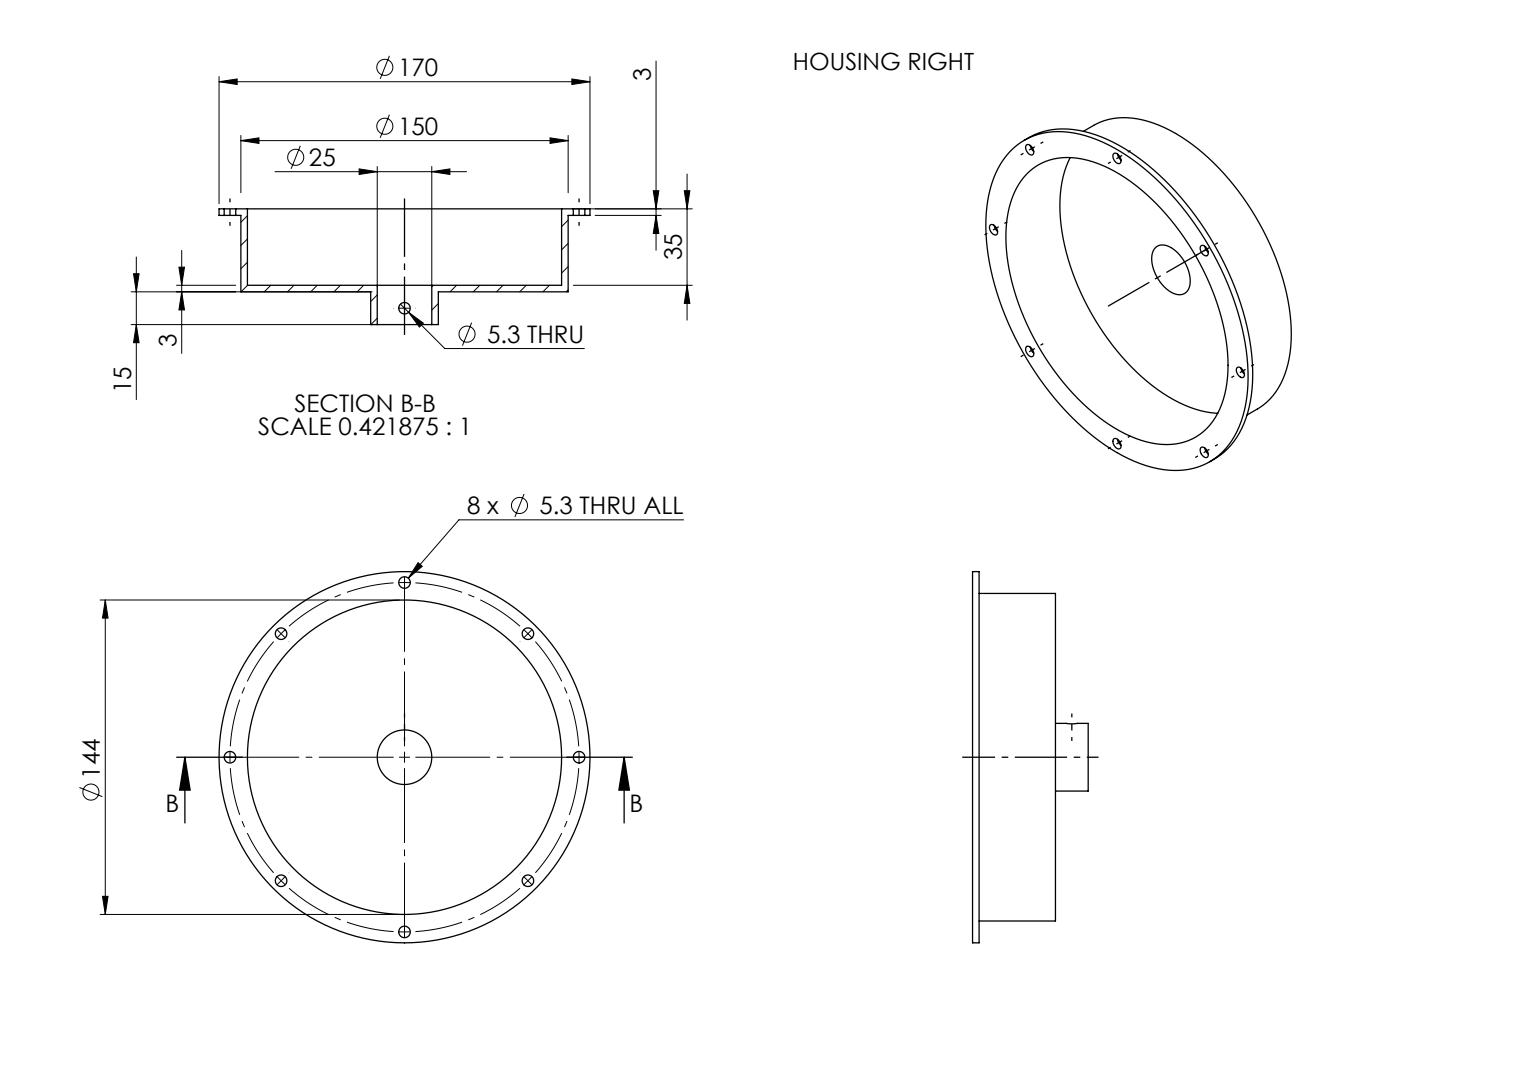
ISO-10303-21;
HEADER;
FILE_DESCRIPTION (('STEP AP214'),
    '1' );
FILE_NAME ('housing right.step',
    '2026-10-08T08:02:49',
    ( '' ),
    ( '' ),
    'SwSTEP 2.0',
    'SolidWorks 2026',
    '' );
FILE_SCHEMA (( 'AUTOMOTIVE_DESIGN' ));
ENDSEC;

DATA;
#5=FACE_OUTER_BOUND ( 'NONE', #24544, .T. ) ;
#96=VERTEX_POINT ( 'NONE', #35469 ) ;
#191=CARTESIAN_POINT ( 'NONE',  ( 52.60669624972128844, 15.41611702489417723, 1.616806307337775861 ) ) ;
#231=ORIENTED_EDGE ( 'NONE', *, *, #52615, .T. ) ;
#243=VERTEX_POINT ( 'NONE', #51378 ) ;
#255=ORIENTED_EDGE ( 'NONE', *, *, #39405, .T. ) ;
#274=COLOUR_RGB ( '', 0.66274510, 0.83137255, 0.94901961) ;
#323=DIRECTION ( 'NONE',  ( -1.000000000000000000, -5.380183451256670742E-17, 1.298891185607911324E-16 ) ) ;
#362=SHAPE_REPRESENTATION ( 'housing right', ( #14677 ), #14881 ) ;
#449=AXIS2_PLACEMENT_3D ( 'NONE', #23041, #9232, #46861 ) ;
#451=EDGE_CURVE ( 'NONE', #48858, #40875, #52468, .T. ) ;
#522=FACE_OUTER_BOUND ( 'NONE', #7239, .T. ) ;
#540=CARTESIAN_POINT ( 'NONE',  ( 52.25260954720639006, 15.37154784856826772, -1.995153943981983202 ) ) ;
#572=CARTESIAN_POINT ( 'NONE',  ( 5.000000000000007994, -58.44237546506767700, -54.69470952477997372 ) ) ;
#620=ORIENTED_EDGE ( 'NONE', *, *, #5146, .T. ) ;
#650=AXIS2_PLACEMENT_3D ( 'NONE', #4623, #9354, #47896 ) ;
#673=CARTESIAN_POINT ( 'NONE',  ( 8.000000000000007105, -56.56854249492331377, -56.56854249492430142 ) ) ;
#689=AXIS2_PLACEMENT_3D ( 'NONE', #15589, #28433, #47560 ) ;
#696=DIRECTION ( 'NONE',  ( -1.000000000000000000, -1.836909530733580185E-16, 1.836909530733574022E-16 ) ) ;
#702=EDGE_LOOP ( 'NONE', ( #10491, #19240, #32643, #32157 ) ) ;
#735=CIRCLE ( 'NONE', #51752, 2.649999999999997691 ) ;
#816=DIRECTION ( 'NONE',  ( 0.000000000000000000, 0.7071067811865527908, -0.7071067811865421326 ) ) ;
#915=AXIS2_PLACEMENT_3D ( 'NONE', #38595, #48285, #43928 ) ;
#936=CARTESIAN_POINT ( 'NONE',  ( 4.999999999999997335, 9.184547653667864935E-16, -9.629649721936170507E-32 ) ) ;
#958=DIRECTION ( 'NONE',  ( 0.000000000000000000, -0.7071067811865487940, 0.7071067811865461294 ) ) ;
#1011=ORIENTED_EDGE ( 'NONE', *, *, #3651, .F. ) ;
#1013=CARTESIAN_POINT ( 'NONE',  ( 50.50000000000000000, 0.000000000000000000, -2.649999999999992806 ) ) ;
#1079=EDGE_CURVE ( 'NONE', #57986, #43044, #10426, .T. ) ;
#1087=EDGE_LOOP ( 'NONE', ( #1602, #31859, #25371, #6168 ) ) ;
#1113=FACE_OUTER_BOUND ( 'NONE', #4513, .T. ) ;
#1258=CARTESIAN_POINT ( 'NONE',  ( 43.00000000000000000, -15.49999999999999645, -2.995852231480067093E-16 ) ) ;
#1274=DIRECTION ( 'NONE',  ( -1.000000000000000000, -1.836909530733573776E-16, 1.925929944387235853E-32 ) ) ;
#1387=DIRECTION ( 'NONE',  ( 0.000000000000000000, 0.000000000000000000, 1.000000000000000000 ) ) ;
#1485=ORIENTED_EDGE ( 'NONE', *, *, #15585, .F. ) ;
#1568=CARTESIAN_POINT ( 'NONE',  ( 52.88125656235560967, 12.44562621623030374, 1.175754242111713532 ) ) ;
#1596=FACE_BOUND ( 'NONE', #57316, .T. ) ;
#1602=ORIENTED_EDGE ( 'NONE', *, *, #33800, .T. ) ;
#1605=ORIENTED_EDGE ( 'NONE', *, *, #37368, .F. ) ;
#1646=EDGE_CURVE ( 'NONE', #14994, #48858, #28079, .T. ) ;
#1654=DIRECTION ( 'NONE',  ( -1.000000000000000000, -3.673819061467147552E-16, 1.925929944387235306E-32 ) ) ;
#1658=AXIS2_PLACEMENT_3D ( 'NONE', #1806, #16240, #49131 ) ;
#1757=CIRCLE ( 'NONE', #29764, 2.649999999999999467 ) ;
#1773=DIRECTION ( 'NONE',  ( -1.000000000000000000, -1.836909530733573776E-16, 1.925929944387235853E-32 ) ) ;
#1778=AXIS2_PLACEMENT_3D ( 'NONE', #20254, #15546, #816 ) ;
#1806=CARTESIAN_POINT ( 'NONE',  ( 5.000000000000007994, -56.56854249492410958, 56.56854249492351983 ) ) ;
#1810=VECTOR ( 'NONE', #7131, 1000.000000000000000 ) ;
#1818=FILL_AREA_STYLE_COLOUR ( '', #25853 ) ;
#1858=VERTEX_POINT ( 'NONE', #34439 ) ;
#1883=CARTESIAN_POINT ( 'NONE',  ( 52.61790645059762284, 12.39576633866792044, -1.629651744153580939 ) ) ;
#1887=VERTEX_POINT ( 'NONE', #36294 ) ;
#1938=VECTOR ( 'NONE', #21205, 1000.000000000000000 ) ;
#1939=CARTESIAN_POINT ( 'NONE',  ( 49.80403646751975799, 12.23154873426529399, 2.580195994037977059 ) ) ;
#2014=LINE ( 'NONE', #30525, #29451 ) ;
#2018=ORIENTED_EDGE ( 'NONE', *, *, #8269, .F. ) ;
#2024=CYLINDRICAL_SURFACE ( 'NONE', #46927, 2.649999999999992806 ) ;
#2160=AXIS2_PLACEMENT_3D ( 'NONE', #3680, #4593, #22815 ) ;
#2183=CARTESIAN_POINT ( 'NONE',  ( 51.83055647397077337, 12.28729589684768264, 2.298227778111301856 ) ) ;
#2186=ORIENTED_EDGE ( 'NONE', *, *, #37368, .T. ) ;
#2360=EDGE_CURVE ( 'NONE', #6447, #24288, #28038, .T. ) ;
#2369=FACE_OUTER_BOUND ( 'NONE', #43922, .T. ) ;
#2380=AXIS2_PLACEMENT_3D ( 'NONE', #47153, #47762, #5118 ) ;
#2435=( NAMED_UNIT ( * ) PLANE_ANGLE_UNIT ( ) SI_UNIT ( $, .RADIAN. ) );
#2488=DIRECTION ( 'NONE',  ( -1.000000000000000000, -3.673819061467147552E-16, 1.925929944387235306E-32 ) ) ;
#2499=CARTESIAN_POINT ( 'NONE',  ( 4.999999999999986677, 56.56854249492450037, -56.56854249492312192 ) ) ;
#2514=CARTESIAN_POINT ( 'NONE',  ( 5.000000000000010658, -72.00000000000002842, 8.817456953860946444E-15 ) ) ;
#2520=DIRECTION ( 'NONE',  ( 0.000000000000000000, 0.000000000000000000, -1.000000000000000000 ) ) ;
#2558=CARTESIAN_POINT ( 'NONE',  ( 50.50000000000000000, 12.21587082446438011, -2.649999999999992806 ) ) ;
#2661=CARTESIAN_POINT ( 'NONE',  ( 7.999999999999981348, 85.00000000000001421, 1.040949779275250495E-14 ) ) ;
#2744=SHAPE_REPRESENTATION_RELATIONSHIP ( 'NONE' , 'NONE' ,  #362, #34065 ) ;
#2748=CARTESIAN_POINT ( 'NONE',  ( 5.000000000000007994, -54.69470952477976056, 58.44237546506787595 ) ) ;
#2759=APPLICATION_CONTEXT ( 'automotive_design' ) ;
#2822=AXIS2_PLACEMENT_3D ( 'NONE', #46688, #22564, #41688 ) ;
#2939=CIRCLE ( 'NONE', #47947, 72.00000000000002842 ) ;
#2960=DIRECTION ( 'NONE',  ( -1.000000000000000000, -1.836909530733580185E-16, 1.836909530733574022E-16 ) ) ;
#3095=ORIENTED_EDGE ( 'NONE', *, *, #9104, .T. ) ;
#3162=ORIENTED_EDGE ( 'NONE', *, *, #6685, .T. ) ;
#3253=CARTESIAN_POINT ( 'NONE',  ( 7.999999999999986677, 56.56854249492371878, 56.56854249492391062 ) ) ;
#3375=DIRECTION ( 'NONE',  ( -1.850371707708593823E-16, 1.000000000000000000, 0.000000000000000000 ) ) ;
#3377=EDGE_LOOP ( 'NONE', ( #255, #7217 ) ) ;
#3435=CARTESIAN_POINT ( 'NONE',  ( 7.999999999999996447, -2.778489794828638662E-13, 80.00000000000001421 ) ) ;
#3442=ORIENTED_EDGE ( 'NONE', *, *, #8024, .T. ) ;
#3459=EDGE_CURVE ( 'NONE', #1887, #50598, #34882, .T. ) ;
#3517=ORIENTED_EDGE ( 'NONE', *, *, #21854, .T. ) ;
#3543=DIRECTION ( 'NONE',  ( 1.000000000000000000, 1.836909530733573776E-16, -1.925929944387235853E-32 ) ) ;
#3646=CYLINDRICAL_SURFACE ( 'NONE', #22822, 2.649999999999992806 ) ;
#3651=EDGE_CURVE ( 'NONE', #25227, #26701, #35913, .T. ) ;
#3663=SURFACE_STYLE_FILL_AREA ( #20946 ) ;
#3680=CARTESIAN_POINT ( 'NONE',  ( 50.50000000000000000, 0.000000000000000000, 0.000000000000000000 ) ) ;
#3688=ORIENTED_EDGE ( 'NONE', *, *, #12608, .T. ) ;
#3750=CARTESIAN_POINT ( 'NONE',  ( 5.000000000000007994, -56.56854249492331377, -56.56854249492430142 ) ) ;
#3759=CARTESIAN_POINT ( 'NONE',  ( 0.000000000000000000, 0.000000000000000000, 0.000000000000000000 ) ) ;
#3771=PRODUCT_DEFINITION ( 'UNKNOWN', '', #29877, #38625 ) ;
#3868=EDGE_CURVE ( 'NONE', #59695, #9789, #28867, .T. ) ;
#3988=DIRECTION ( 'NONE',  ( 1.000000000000000000, 1.836909530733573776E-16, -1.925929944387235853E-32 ) ) ;
#4013=ORIENTED_EDGE ( 'NONE', *, *, #28082, .F. ) ;
#4029=CYLINDRICAL_SURFACE ( 'NONE', #41805, 2.649999999999992806 ) ;
#4130=CARTESIAN_POINT ( 'NONE',  ( 4.999999999999997335, 9.184547653667862963E-16, -9.629649721936174886E-32 ) ) ;
#4147=DIRECTION ( 'NONE',  ( 0.000000000000000000, 0.000000000000000000, 1.000000000000000000 ) ) ;
#4151=ORIENTED_EDGE ( 'NONE', *, *, #33324, .F. ) ;
#4178=VERTEX_POINT ( 'NONE', #46032 ) ;
#4336=CARTESIAN_POINT ( 'NONE',  ( 48.39278666958532682, 15.41618682757451353, 1.616172141987365363 ) ) ;
#4381=CYLINDRICAL_SURFACE ( 'NONE', #50819, 75.00000000000001421 ) ;
#4513=EDGE_LOOP ( 'NONE', ( #27565, #49130, #52774, #5751 ) ) ;
#4525=FILL_AREA_STYLE ('',( #27429 ) ) ;
#4593=DIRECTION ( 'NONE',  ( -0.000000000000000000, -1.000000000000000000, -0.000000000000000000 ) ) ;
#4602=AXIS2_PLACEMENT_3D ( 'NONE', #19390, #61048, #61651 ) ;
#4623=CARTESIAN_POINT ( 'NONE',  ( 4.999999999999983125, 80.00000000000001421, -3.562970397116383044E-32 ) ) ;
#4633=CARTESIAN_POINT ( 'NONE',  ( 4.999999999999997335, 8.388739760877188892E-13, -80.00000000000001421 ) ) ;
#4691=AXIS2_PLACEMENT_3D ( 'NONE', #16594, #60110, #25989 ) ;
#4729=DIRECTION ( 'NONE',  ( 1.836766033387207149E-16, -1.000000000000000000, 0.000000000000000000 ) ) ;
#4788=AXIS2_PLACEMENT_3D ( 'NONE', #11876, #22481, #36916 ) ;
#4875=VERTEX_POINT ( 'NONE', #35777 ) ;
#4906=CIRCLE ( 'NONE', #24969, 2.649999999999997691 ) ;
#4930=CARTESIAN_POINT ( 'NONE',  ( 52.60613790598473116, 15.41603472375467909, -1.617730826299683899 ) ) ;
#4957=DIRECTION ( 'NONE',  ( -1.000000000000000000, -1.836909530733554547E-16, -1.836909530733573529E-16 ) ) ;
#5062=EDGE_LOOP ( 'NONE', ( #29514, #1605 ) ) ;
#5118=DIRECTION ( 'NONE',  ( 0.000000000000000000, 0.7071067811865527908, -0.7071067811865421326 ) ) ;
#5129=EDGE_CURVE ( 'NONE', #55350, #25443, #29738, .T. ) ;
#5146=EDGE_CURVE ( 'NONE', #48858, #14994, #26953, .T. ) ;
#5265=FACE_OUTER_BOUND ( 'NONE', #41410, .T. ) ;
#5329=CIRCLE ( 'NONE', #54330, 85.00000000000001421 ) ;
#5399=CARTESIAN_POINT ( 'NONE',  ( 7.999999999999996447, 8.394250489469390599E-13, -80.00000000000001421 ) ) ;
#5405=ORIENTED_EDGE ( 'NONE', *, *, #2360, .T. ) ;
#5468=AXIS2_PLACEMENT_3D ( 'NONE', #18420, #23729, #23419 ) ;
#5523=DIRECTION ( 'NONE',  ( -1.000000000000000000, -1.836909530733580185E-16, 1.836909530733574022E-16 ) ) ;
#5527=DIRECTION ( 'NONE',  ( 0.000000000000000000, -1.000000000000000000, 0.000000000000000000 ) ) ;
#5536=CARTESIAN_POINT ( 'NONE',  ( 52.88193763142881210, 15.45628894957374655, -1.174165929033795353 ) ) ;
#5751=ORIENTED_EDGE ( 'NONE', *, *, #6356, .T. ) ;
#5912=ORIENTED_EDGE ( 'NONE', *, *, #55151, .T. ) ;
#5918=ORIENTED_EDGE ( 'NONE', *, *, #2360, .F. ) ;
#5933=EDGE_LOOP ( 'NONE', ( #25583, #3095, #57007, #56092 ) ) ;
#5945=CARTESIAN_POINT ( 'NONE',  ( 52.49662775218939714, 12.37736723654698068, 1.751076765323000828 ) ) ;
#6168=ORIENTED_EDGE ( 'NONE', *, *, #45409, .F. ) ;
#6189=( NAMED_UNIT ( * ) SI_UNIT ( $, .STERADIAN. ) SOLID_ANGLE_UNIT ( ) );
#6210=EDGE_CURVE ( 'NONE', #50555, #49238, #25827, .T. ) ;
#6259=CARTESIAN_POINT ( 'NONE',  ( 58.00000000000000000, 15.50000000000000888, 1.598617315530390651E-15 ) ) ;
#6262=EDGE_CURVE ( 'NONE', #29773, #12923, #17251, .T. ) ;
#6335=LINE ( 'NONE', #54266, #37437 ) ;
#6356=EDGE_CURVE ( 'NONE', #9789, #59695, #14849, .T. ) ;
#6405=CARTESIAN_POINT ( 'NONE',  ( 39.99999999999998579, 72.00000000000004263, -4.333342374871279794E-31 ) ) ;
#6447=VERTEX_POINT ( 'NONE', #17435 ) ;
#6452=ORIENTED_EDGE ( 'NONE', *, *, #54819, .T. ) ;
#6535=ORIENTED_EDGE ( 'NONE', *, *, #18753, .T. ) ;
#6559=CARTESIAN_POINT ( 'NONE',  ( 51.18761205055119490, 12.23403309190988075, -2.565078866171123906 ) ) ;
#6561=EDGE_CURVE ( 'NONE', #16220, #6447, #22842, .T. ) ;
#6604=ORIENTED_EDGE ( 'NONE', *, *, #44026, .T. ) ;
#6663=CARTESIAN_POINT ( 'NONE',  ( 7.999999999999996447, -2.650000000000270806, 80.00000000000000000 ) ) ;
#6685=EDGE_CURVE ( 'NONE', #8457, #243, #58819, .T. ) ;
#6752=AXIS2_PLACEMENT_3D ( 'NONE', #21935, #59825, #26941 ) ;
#6776=ORIENTED_EDGE ( 'NONE', *, *, #49614, .F. ) ;
#6792=ORIENTED_EDGE ( 'NONE', *, *, #18019, .T. ) ;
#6906=CIRCLE ( 'NONE', #31942, 2.649999999999997691 ) ;
#6910=ADVANCED_FACE ( 'NONE', ( #28217 ), #4381, .T. ) ;
#7103=EDGE_LOOP ( 'NONE', ( #32035, #49413, #2186, #46245 ) ) ;
#7131=DIRECTION ( 'NONE',  ( -1.000000000000000000, -3.135800716341471541E-16, -1.298891185607920445E-16 ) ) ;
#7166=CIRCLE ( 'NONE', #44250, 75.00000000000001421 ) ;
#7217=ORIENTED_EDGE ( 'NONE', *, *, #9358, .T. ) ;
#7239=EDGE_LOOP ( 'NONE', ( #4013, #45371, #9473, #45138, #17668, #60804, #13702 ) ) ;
#7248=ORIENTED_EDGE ( 'NONE', *, *, #9104, .F. ) ;
#7252=AXIS2_PLACEMENT_3D ( 'NONE', #46444, #18538, #41751 ) ;
#7318=FACE_OUTER_BOUND ( 'NONE', #43411, .T. ) ;
#7362=EDGE_LOOP ( 'NONE', ( #28161, #35366 ) ) ;
#7366=CARTESIAN_POINT ( 'NONE',  ( 4.999999999999997335, 9.184547653667864935E-16, -9.629649721936170507E-32 ) ) ;
#7418=CARTESIAN_POINT ( 'NONE',  ( 8.000000000000007105, -56.56854249492331377, -56.56854249492430142 ) ) ;
#7424=ORIENTED_EDGE ( 'NONE', *, *, #9041, .F. ) ;
#7460=VECTOR ( 'NONE', #50221, 1000.000000000000000 ) ;
#7471=CARTESIAN_POINT ( 'NONE',  ( 5.000000000000013323, -85.00000000000001421, -9.629649721936174886E-32 ) ) ;
#7492=VECTOR ( 'NONE', #43754, 1000.000000000000000 ) ;
#7504=ORIENTED_EDGE ( 'NONE', *, *, #22869, .F. ) ;
#7537=FACE_OUTER_BOUND ( 'NONE', #45126, .T. ) ;
#7552=ORIENTED_EDGE ( 'NONE', *, *, #43108, .T. ) ;
#7686=DIRECTION ( 'NONE',  ( -1.836909530733573776E-16, 1.000000000000000000, 0.000000000000000000 ) ) ;
#7765=PRODUCT ( 'housing right', 'housing right', '', ( #12722 ) ) ;
#7842=DIRECTION ( 'NONE',  ( 1.000000000000000000, 1.836909530733573776E-16, -1.925929944387235853E-32 ) ) ;
#8024=EDGE_CURVE ( 'NONE', #25443, #22251, #31564, .T. ) ;
#8185=CARTESIAN_POINT ( 'NONE',  ( 50.15117465005047137, 12.21965674021488368, -2.632719331364402393 ) ) ;
#8192=ORIENTED_EDGE ( 'NONE', *, *, #38584, .F. ) ;
#8232=ORIENTED_EDGE ( 'NONE', *, *, #54819, .F. ) ;
#8233=DIRECTION ( 'NONE',  ( -1.000000000000000000, -5.380183451256670742E-17, 1.298891185607911324E-16 ) ) ;
#8259=ORIENTED_EDGE ( 'NONE', *, *, #9041, .T. ) ;
#8269=EDGE_CURVE ( 'NONE', #29773, #54373, #53933, .T. ) ;
#8444=DIRECTION ( 'NONE',  ( 0.000000000000000000, 1.000000000000000000, 0.000000000000000000 ) ) ;
#8457=VERTEX_POINT ( 'NONE', #42351 ) ;
#8487=FACE_OUTER_BOUND ( 'NONE', #10114, .T. ) ;
#8569=AXIS2_PLACEMENT_3D ( 'NONE', #936, #23828, #33241 ) ;
#8609=AXIS2_PLACEMENT_3D ( 'NONE', #29297, #48408, #14919 ) ;
#8680=CARTESIAN_POINT ( 'NONE',  ( 52.25008115675156972, 15.37124894287441279, 1.997531998838311784 ) ) ;
#8691=DIRECTION ( 'NONE',  ( 1.000000000000000000, 1.836909530733573776E-16, -1.925929944387235853E-32 ) ) ;
#8716=CARTESIAN_POINT ( 'NONE',  ( 4.999999999999997335, 8.388739760877188892E-13, -80.00000000000001421 ) ) ;
#8771=CARTESIAN_POINT ( 'NONE',  ( 8.000000000000007105, -58.44237546506767700, -54.69470952477997372 ) ) ;
#8776=AXIS2_PLACEMENT_3D ( 'NONE', #7366, #21488, #59694 ) ;
#8848=CYLINDRICAL_SURFACE ( 'NONE', #35618, 85.00000000000001421 ) ;
#8861=EDGE_CURVE ( 'NONE', #12452, #23359, #2014, .T. ) ;
#9026=CARTESIAN_POINT ( 'NONE',  ( 53.01412262506746487, 15.47721078833569841, -0.8552660025069994676 ) ) ;
#9041=EDGE_CURVE ( 'NONE', #15197, #37408, #42738, .T. ) ;
#9065=CARTESIAN_POINT ( 'NONE',  ( 48.74902663329513786, 15.37135949308304816, 1.996608280103705058 ) ) ;
#9104=EDGE_CURVE ( 'NONE', #22095, #22251, #38658, .T. ) ;
#9135=ORIENTED_EDGE ( 'NONE', *, *, #48508, .F. ) ;
#9145=CARTESIAN_POINT ( 'NONE',  ( 50.50000000000000000, 15.27178771460631168, -2.649999999999992806 ) ) ;
#9196=DIRECTION ( 'NONE',  ( 0.000000000000000000, -1.047444401652941269E-14, 1.000000000000000000 ) ) ;
#9222=EDGE_LOOP ( 'NONE', ( #6535, #46586 ) ) ;
#9232=DIRECTION ( 'NONE',  ( 1.000000000000000000, 1.836909530733573776E-16, -1.925929944387235853E-32 ) ) ;
#9295=ORIENTED_EDGE ( 'NONE', *, *, #33396, .T. ) ;
#9302=CARTESIAN_POINT ( 'NONE',  ( 53.06470156691138129, 15.48560858660915507, 0.6891024955566218413 ) ) ;
#9314=CARTESIAN_POINT ( 'NONE',  ( 50.32467004767242713, 15.27178771460630635, -2.649999999999991918 ) ) ;
#9339=EDGE_CURVE ( 'NONE', #49193, #29142, #52340, .T. ) ;
#9354=DIRECTION ( 'NONE',  ( -1.000000000000000000, -0.000000000000000000, 1.925929944387235853E-32 ) ) ;
#9358=EDGE_CURVE ( 'NONE', #22596, #20457, #26502, .T. ) ;
#9367=ORIENTED_EDGE ( 'NONE', *, *, #22995, .F. ) ;
#9473=ORIENTED_EDGE ( 'NONE', *, *, #451, .T. ) ;
#9529=DIRECTION ( 'NONE',  ( 0.000000000000000000, 0.000000000000000000, -1.000000000000000000 ) ) ;
#9535=APPLICATION_CONTEXT ( 'automotive_design' ) ;
#9621=EDGE_LOOP ( 'NONE', ( #48967, #45953 ) ) ;
#9625=CARTESIAN_POINT ( 'NONE',  ( 50.15149541334723438, 15.27480702088406694, -2.632769263815124994 ) ) ;
#9720=FACE_BOUND ( 'NONE', #40678, .T. ) ;
#9789=VERTEX_POINT ( 'NONE', #43524 ) ;
#9848=EDGE_CURVE ( 'NONE', #26701, #25227, #25509, .T. ) ;
#9962=ORIENTED_EDGE ( 'NONE', *, *, #60027, .T. ) ;
#9966=CARTESIAN_POINT ( 'NONE',  ( 51.35572961735444153, 15.29490605596151553, -2.514040278272794637 ) ) ;
#9971=FACE_BOUND ( 'NONE', #15664, .T. ) ;
#9990=VERTEX_POINT ( 'NONE', #37206 ) ;
#9996=ORIENTED_EDGE ( 'NONE', *, *, #3868, .F. ) ;
#10003=ADVANCED_FACE ( 'NONE', ( #46598 ), #3646, .F. ) ;
#10114=EDGE_LOOP ( 'NONE', ( #1485, #33255, #6452, #29907 ) ) ;
#10122=CARTESIAN_POINT ( 'NONE',  ( 48.88249858120726543, 12.32166152761977429, 2.106239978570320304 ) ) ;
#10185=( NAMED_UNIT ( * ) PLANE_ANGLE_UNIT ( ) SI_UNIT ( $, .RADIAN. ) );
#10349=FACE_BOUND ( 'NONE', #25658, .T. ) ;
#10385=B_SPLINE_CURVE_WITH_KNOTS ( 'NONE', 3,
 ( #37601, #61357, #38524, #22865, #61061, #18474, #13793, #32897, #9065, #47288, #4336, #18795, #37921, #34132, #35058, #35368, #40086, #34434 ),
 .UNSPECIFIED., .F., .F.,
 ( 4, 2, 2, 2, 2, 2, 2, 2, 4 ),
 ( 0.008300350213780812239, 0.008819185130678563675, 0.009338020047576315111, 0.009856854964474064812, 0.01037568988137181625, 0.01089452479826956768, 0.01141335971516731912, 0.01193219463206507056, 0.01245102954896282026 ),
 .UNSPECIFIED. ) ;
#10426=LINE ( 'NONE', #24830, #18072 ) ;
#10491=ORIENTED_EDGE ( 'NONE', *, *, #1079, .F. ) ;
#10532=CARTESIAN_POINT ( 'NONE',  ( 40.00000000000000000, 7.347638122934295104E-15, -7.703719777548943412E-31 ) ) ;
#10550=ADVANCED_FACE ( 'NONE', ( #61064 ), #53888, .T. ) ;
#10568=CARTESIAN_POINT ( 'NONE',  ( 4.999999999999986677, 54.69470952478017267, -58.44237546506749936 ) ) ;
#10979=CARTESIAN_POINT ( 'NONE',  ( 4.999999999999998224, -2.649999999999161471, -80.00000000000004263 ) ) ;
#10987=EDGE_LOOP ( 'NONE', ( #14158, #38902, #31865, #59387 ) ) ;
#11005=CARTESIAN_POINT ( 'NONE',  ( 51.35620144615297988, 12.24479674684753761, -2.513874600954978167 ) ) ;
#11054=CLOSED_SHELL ( 'NONE', ( #16134, #10550, #43383, #44525, #10003, #33207, #22022, #53580, #21743, #61635, #57359, #12192, #56573, #6910, #14160, #21274, #61922, #39300, #56281, #22127, #57051, #53773, #44022, #56991, #18338, #61290, #18801, #33471, #55309, #46488, #45799, #21069, #49011 ) ) ;
#11059=DIRECTION ( 'NONE',  ( -0.000000000000000000, -1.000000000000000000, -0.000000000000000000 ) ) ;
#11203=PLANE ( 'NONE',  #45538 ) ;
#11240=( LENGTH_UNIT ( ) NAMED_UNIT ( * ) SI_UNIT ( .MILLI., .METRE. ) );
#11292=ORIENTED_EDGE ( 'NONE', *, *, #22869, .T. ) ;
#11301=CARTESIAN_POINT ( 'NONE',  ( 53.14993166107466749, 12.49998551214889808, -0.1744414439710397502 ) ) ;
#11474=DIRECTION ( 'NONE',  ( 0.000000000000000000, 0.000000000000000000, 1.000000000000000000 ) ) ;
#11504=LINE ( 'NONE', #49703, #1938 ) ;
#11591=ORIENTED_EDGE ( 'NONE', *, *, #39069, .F. ) ;
#11764=CIRCLE ( 'NONE', #59771, 2.649999999999985700 ) ;
#11819=EDGE_LOOP ( 'NONE', ( #33452, #27207, #61717, #49182, #46180 ) ) ;
#11831=EDGE_CURVE ( 'NONE', #33073, #1887, #46628, .T. ) ;
#11848=EDGE_CURVE ( 'NONE', #49193, #29773, #27107, .T. ) ;
#11876=CARTESIAN_POINT ( 'NONE',  ( 4.999999999999983125, 80.00000000000001421, -3.562970397116383044E-32 ) ) ;
#11887=CARTESIAN_POINT ( 'NONE',  ( 5.000000000000007994, -54.69470952477895764, -58.44237546506863623 ) ) ;
#12002=CARTESIAN_POINT ( 'NONE',  ( 50.50000000000000000, 12.21587082446438011, -2.649999999999992806 ) ) ;
#12004=DIRECTION ( 'NONE',  ( -1.000000000000000000, -1.836909530733554547E-16, -1.836909530733573529E-16 ) ) ;
#12036=CARTESIAN_POINT ( 'NONE',  ( 4.999999999999986677, 56.56854249492371878, 56.56854249492391062 ) ) ;
#12040=LINE ( 'NONE', #12648, #7460 ) ;
#12110=SHAPE_DEFINITION_REPRESENTATION ( #50273, #362 ) ;
#12192=ADVANCED_FACE ( 'NONE', ( #2369 ), #21809, .F. ) ;
#12247=LINE ( 'NONE', #40159, #30933 ) ;
#12428=AXIS2_PLACEMENT_3D ( 'NONE', #25100, #1274, #39536 ) ;
#12452=VERTEX_POINT ( 'NONE', #6663 ) ;
#12520=DIRECTION ( 'NONE',  ( 0.000000000000000000, 0.7071067811865395791, 0.7071067811865553443 ) ) ;
#12608=EDGE_CURVE ( 'NONE', #61948, #59796, #34720, .T. ) ;
#12648=CARTESIAN_POINT ( 'NONE',  ( 4.999999999999986677, 58.44237546506882808, -54.69470952477875869 ) ) ;
#12653=ORIENTED_EDGE ( 'NONE', *, *, #54361, .T. ) ;
#12681=DIRECTION ( 'NONE',  ( 1.850371707708593823E-16, -1.000000000000000000, 0.000000000000000000 ) ) ;
#12722=PRODUCT_CONTEXT ( 'NONE', #9535, 'mechanical' ) ;
#12806=DIRECTION ( 'NONE',  ( -1.000000000000000000, -1.836909530733573776E-16, 1.103352205049209901E-32 ) ) ;
#12834=CARTESIAN_POINT ( 'NONE',  ( 4.999999999999986677, 56.56854249492450037, -56.56854249492312192 ) ) ;
#12880=CARTESIAN_POINT ( 'NONE',  ( 43.00000000000000000, 5.682605120120046040E-15, -2.995852231480065614E-16 ) ) ;
#12895=CARTESIAN_POINT ( 'NONE',  ( 4.999999999999997335, 9.184547653667864935E-16, -9.629649721936170507E-32 ) ) ;
#12923=VERTEX_POINT ( 'NONE', #60160 ) ;
#12933=CYLINDRICAL_SURFACE ( 'NONE', #38608, 2.649999999999992806 ) ;
#12952=DIRECTION ( 'NONE',  ( 0.000000000000000000, 0.000000000000000000, -1.000000000000000000 ) ) ;
#13009=DIRECTION ( 'NONE',  ( 0.000000000000000000, -0.7071067811865461294, -0.7071067811865487940 ) ) ;
#13023=CARTESIAN_POINT ( 'NONE',  ( 8.000000000000012434, -80.00000000000001421, 2.649999999999992806 ) ) ;
#13040=EDGE_LOOP ( 'NONE', ( #29972, #17063 ) ) ;
#13095=ORIENTED_EDGE ( 'NONE', *, *, #28488, .T. ) ;
#13104=( NAMED_UNIT ( * ) PLANE_ANGLE_UNIT ( ) SI_UNIT ( $, .RADIAN. ) );
#13136=ORIENTED_EDGE ( 'NONE', *, *, #31544, .T. ) ;
#13366=CARTESIAN_POINT ( 'NONE',  ( 7.999999999999996447, -2.778489794828638662E-13, 80.00000000000001421 ) ) ;
#13415=LINE ( 'NONE', #22496, #19236 ) ;
#13477=AXIS2_PLACEMENT_3D ( 'NONE', #12834, #13760, #12520 ) ;
#13702=ORIENTED_EDGE ( 'NONE', *, *, #6262, .T. ) ;
#13760=DIRECTION ( 'NONE',  ( -1.000000000000000000, -5.380183451256491399E-17, -1.298891185607892835E-16 ) ) ;
#13788=CIRCLE ( 'NONE', #48771, 2.649999999999985700 ) ;
#13793=CARTESIAN_POINT ( 'NONE',  ( 49.17116576101606995, 15.32881676279135874, 2.299327193150783266 ) ) ;
#13822=DIRECTION ( 'NONE',  ( 1.000000000000000000, 0.000000000000000000, 0.000000000000000000 ) ) ;
#13900=VERTEX_POINT ( 'NONE', #2748 ) ;
#13988=CARTESIAN_POINT ( 'NONE',  ( 58.00000000000000000, 0.000000000000000000, 12.50000000000000000 ) ) ;
#14062=CARTESIAN_POINT ( 'NONE',  ( 53.14999999999999858, 15.50000000000000711, 1.598617295522242905E-15 ) ) ;
#14081=CYLINDRICAL_SURFACE ( 'NONE', #650, 2.649999999999992806 ) ;
#14136=ORIENTED_EDGE ( 'NONE', *, *, #54361, .F. ) ;
#14139=FACE_BOUND ( 'NONE', #43742, .T. ) ;
#14158=ORIENTED_EDGE ( 'NONE', *, *, #44026, .F. ) ;
#14160=ADVANCED_FACE ( 'NONE', ( #35215 ), #57746, .T. ) ;
#14198=ORIENTED_EDGE ( 'NONE', *, *, #61572, .F. ) ;
#14236=LINE ( 'NONE', #18937, #28561 ) ;
#14290=DIRECTION ( 'NONE',  ( -1.000000000000000000, -1.836909530733573776E-16, 1.925929944387235853E-32 ) ) ;
#14309=EDGE_LOOP ( 'NONE', ( #7424, #50025, #6792, #52169 ) ) ;
#14338=CARTESIAN_POINT ( 'NONE',  ( 51.35430322215398746, 15.29482815186059774, 2.514508868274447639 ) ) ;
#14577=ORIENTED_EDGE ( 'NONE', *, *, #451, .F. ) ;
#14597=CARTESIAN_POINT ( 'NONE',  ( 58.00000000000000000, -15.49999999999999112, -2.995852231480068572E-16 ) ) ;
#14639=CARTESIAN_POINT ( 'NONE',  ( 43.00000000000000000, 15.50000000000000533, 1.598617315530390848E-15 ) ) ;
#14654=EDGE_LOOP ( 'NONE', ( #1011, #59641, #27688, #6776 ) ) ;
#14674=CARTESIAN_POINT ( 'NONE',  ( 53.15000000000000568, 15.50000000000000711, -0.1732459626436144429 ) ) ;
#14677=AXIS2_PLACEMENT_3D ( 'NONE', #3759, #61387, #13822 ) ;
#14724=VERTEX_POINT ( 'NONE', #18187 ) ;
#14824=VECTOR ( 'NONE', #46380, 1000.000000000000000 ) ;
#14849=CIRCLE ( 'NONE', #59853, 2.649999999999997691 ) ;
#14881=( GEOMETRIC_REPRESENTATION_CONTEXT ( 3 ) GLOBAL_UNCERTAINTY_ASSIGNED_CONTEXT ( ( #48012 ) ) GLOBAL_UNIT_ASSIGNED_CONTEXT ( ( #11240, #2435, #6189 ) ) REPRESENTATION_CONTEXT ( 'NONE', 'WORKASPACE' ) );
#14919=DIRECTION ( 'NONE',  ( 0.000000000000000000, -0.7071067811865553443, 0.7071067811865395791 ) ) ;
#14969=CARTESIAN_POINT ( 'NONE',  ( 4.999999999999997335, -2.784000523420839360E-13, 80.00000000000001421 ) ) ;
#14987=AXIS2_PLACEMENT_3D ( 'NONE', #46493, #3543, #42125 ) ;
#14994=VERTEX_POINT ( 'NONE', #45705 ) ;
#15073=ORIENTED_EDGE ( 'NONE', *, *, #32108, .F. ) ;
#15197=VERTEX_POINT ( 'NONE', #32219 ) ;
#15397=CARTESIAN_POINT ( 'NONE',  ( 51.18991377541220800, 12.23415317001104086, 2.564509504438283294 ) ) ;
#15418=CARTESIAN_POINT ( 'NONE',  ( 4.999999999999986677, 56.56854249492450037, -56.56854249492312192 ) ) ;
#15444=CARTESIAN_POINT ( 'NONE',  ( 47.85015878647476484, 12.49996633727064932, 0.3510238927397298925 ) ) ;
#15462=CARTESIAN_POINT ( 'NONE',  ( 8.000000000000007105, -54.69470952477895764, -58.44237546506863623 ) ) ;
#15546=DIRECTION ( 'NONE',  ( -1.000000000000000000, -3.135800716341471541E-16, -1.298891185607920445E-16 ) ) ;
#15585=EDGE_CURVE ( 'NONE', #22596, #50555, #39020, .T. ) ;
#15589=CARTESIAN_POINT ( 'NONE',  ( 40.00000000000000000, 0.000000000000000000, 0.000000000000000000 ) ) ;
#15657=CIRCLE ( 'NONE', #4602, 15.50000000000000000 ) ;
#15664=EDGE_LOOP ( 'NONE', ( #30806, #31931 ) ) ;
#15704=CARTESIAN_POINT ( 'NONE',  ( 50.50000000000000000, 12.21587082446438011, 2.649999999999992806 ) ) ;
#15718=AXIS2_PLACEMENT_3D ( 'NONE', #22657, #43016, #61452 ) ;
#15757=CARTESIAN_POINT ( 'NONE',  ( 48.20159250628719150, 12.42985392437715220, 1.330251472907249433 ) ) ;
#15791=DIRECTION ( 'NONE',  ( -1.000000000000000000, -3.673819061467147552E-16, 1.925929944387235306E-32 ) ) ;
#15863=ORIENTED_EDGE ( 'NONE', *, *, #60454, .T. ) ;
#15904=FACE_BOUND ( 'NONE', #24389, .T. ) ;
#15995=DIRECTION ( 'NONE',  ( -1.000000000000000000, -1.836909530733573529E-16, 1.361838123766461297E-32 ) ) ;
#16012=CARTESIAN_POINT ( 'NONE',  ( 53.01364348093722612, 12.47163566169240845, -0.8566609489383912868 ) ) ;
#16128=DIRECTION ( 'NONE',  ( 0.000000000000000000, 0.000000000000000000, -1.000000000000000000 ) ) ;
#16131=EDGE_CURVE ( 'NONE', #55350, #22095, #7166, .T. ) ;
#16134=ADVANCED_FACE ( 'NONE', ( #17814 ), #42555, .F. ) ;
#16182=ORIENTED_EDGE ( 'NONE', *, *, #28199, .F. ) ;
#16220=VERTEX_POINT ( 'NONE', #43806 ) ;
#16240=DIRECTION ( 'NONE',  ( -1.000000000000000000, -3.135800716341489291E-16, 1.298891185607901956E-16 ) ) ;
#16271=ORIENTED_EDGE ( 'NONE', *, *, #11848, .F. ) ;
#16303=DIRECTION ( 'NONE',  ( 0.000000000000000000, 0.7071067811865382469, 0.7071067811865566766 ) ) ;
#16318=DIRECTION ( 'NONE',  ( -1.000000000000000000, -1.836909530733573776E-16, 1.925929944387235853E-32 ) ) ;
#16496=AXIS2_PLACEMENT_3D ( 'NONE', #38904, #23850, #32959 ) ;
#16538=DIRECTION ( 'NONE',  ( 0.000000000000000000, 0.7071067811865421326, 0.7071067811865527908 ) ) ;
#16581=B_SPLINE_CURVE_WITH_KNOTS ( 'NONE', 3,
 ( #20701, #29783, #39841, #6559, #11005, #58894, #40449, #30703, #49819, #1883, #35126, #16012, #58575, #16623, #11301, #30389, #54184, #59512, #58266, #1568, #53882, #48894, #5945, #26018, #25084, #2183, #44537, #44230, #15397, #54491, #49506, #15704 ),
 .UNSPECIFIED., .F., .F.,
 ( 4, 2, 2, 2, 2, 2, 2, 2, 2, 2, 2, 2, 2, 2, 2, 4 ),
 ( 0.000000000000000000, 0.0005192934025038106532, 0.001038586805007621306, 0.001557880207511431851, 0.002077173610015242613, 0.003115760415022862835, 0.003635053817526677066, 0.004154347220030491297, 0.004673640622534305095, 0.005192934025038119759, 0.005712227427541933557, 0.006231520830045749089, 0.006750814232549562886, 0.007270107635053377551, 0.007789401037557191348, 0.008308694440061006881 ),
 .UNSPECIFIED. ) ;
#16594=CARTESIAN_POINT ( 'NONE',  ( 4.999999999999997335, 9.184547653667864935E-16, -9.629649721936170507E-32 ) ) ;
#16623=CARTESIAN_POINT ( 'NONE',  ( 53.13300907242233251, 12.49636441417896116, -0.3467375140025887870 ) ) ;
#16704=CARTESIAN_POINT ( 'NONE',  ( 58.00000000000000000, 8.437969416220405915E-15, -2.995852231480068572E-16 ) ) ;
#16979=DIRECTION ( 'NONE',  ( -3.273063162220399693E-16, 1.000000000000000000, 1.047380211910527902E-14 ) ) ;
#17059=CARTESIAN_POINT ( 'NONE',  ( 4.999999999999997335, 9.184547653667862963E-16, -9.629649721936174886E-32 ) ) ;
#17063=ORIENTED_EDGE ( 'NONE', *, *, #6210, .F. ) ;
#17070=CYLINDRICAL_SURFACE ( 'NONE', #21765, 12.50000000000000000 ) ;
#17117=DIRECTION ( 'NONE',  ( 1.000000000000000000, 1.836909530733573776E-16, -1.925929944387235853E-32 ) ) ;
#17251=B_SPLINE_CURVE_WITH_KNOTS ( 'NONE', 3,
 ( #28436, #37562, #33787, #47876, #9966, #47253, #43817, #29067, #540, #38485, #4930, #38800, #5536, #9026, #24061, #57539, #14674, #14062 ),
 .UNSPECIFIED., .F., .F.,
 ( 4, 2, 2, 2, 2, 2, 2, 2, 4 ),
 ( 0.000000000000000000, 0.0005188972795902839106, 0.001037794559180567821, 0.001556691838770851623, 0.002075589118361135643, 0.002594486397951419662, 0.003113383677541703247, 0.003632280957131987266, 0.004151178236722271285 ),
 .UNSPECIFIED. ) ;
#17257=CARTESIAN_POINT ( 'NONE',  ( 8.000000000000012434, -80.00000000000001421, -2.147411887991766662E-31 ) ) ;
#17278=CARTESIAN_POINT ( 'NONE',  ( 43.00000000000000000, 0.000000000000000000, 0.000000000000000000 ) ) ;
#17389=DIRECTION ( 'NONE',  ( -1.000000000000000000, -1.836909530733573776E-16, 1.925929944387235853E-32 ) ) ;
#17423=( LENGTH_UNIT ( ) NAMED_UNIT ( * ) SI_UNIT ( .MILLI., .METRE. ) );
#17435=CARTESIAN_POINT ( 'NONE',  ( 7.999999999999986677, 54.69470952477936976, 58.44237546506825964 ) ) ;
#17575=AXIS2_PLACEMENT_3D ( 'NONE', #24916, #35244, #16128 ) ;
#17580=DIRECTION ( 'NONE',  ( -1.807003620809173399E-16, 1.000000000000000000, 0.000000000000000000 ) ) ;
#17650=ORIENTED_EDGE ( 'NONE', *, *, #38858, .T. ) ;
#17668=ORIENTED_EDGE ( 'NONE', *, *, #9339, .F. ) ;
#17737=DIRECTION ( 'NONE',  ( -1.000000000000000000, -3.135800716341489291E-16, 1.298891185607901956E-16 ) ) ;
#17742=CIRCLE ( 'NONE', #4691, 72.00000000000002842 ) ;
#17782=VECTOR ( 'NONE', #18110, 1000.000000000000000 ) ;
#17814=FACE_OUTER_BOUND ( 'NONE', #56413, .T. ) ;
#17874=EDGE_LOOP ( 'NONE', ( #17650, #53176 ) ) ;
#17887=AXIS2_PLACEMENT_3D ( 'NONE', #673, #28883, #19816 ) ;
#17947=EDGE_CURVE ( 'NONE', #22095, #55350, #61278, .T. ) ;
#17982=AXIS2_PLACEMENT_3D ( 'NONE', #22211, #41340, #51310 ) ;
#18007=DIRECTION ( 'NONE',  ( -1.000000000000000000, -5.380183451256670742E-17, 1.298891185607911324E-16 ) ) ;
#18019=EDGE_CURVE ( 'NONE', #96, #50941, #23854, .T. ) ;
#18072=VECTOR ( 'NONE', #696, 1000.000000000000000 ) ;
#18110=DIRECTION ( 'NONE',  ( -1.000000000000000000, -1.836909530733573776E-16, 1.925929944387235579E-32 ) ) ;
#18187=CARTESIAN_POINT ( 'NONE',  ( 50.50000000000000000, 12.21587082446438011, 2.649999999999992806 ) ) ;
#18198=FACE_OUTER_BOUND ( 'NONE', #10987, .T. ) ;
#18270=ORIENTED_EDGE ( 'NONE', *, *, #45409, .T. ) ;
#18338=ADVANCED_FACE ( 'NONE', ( #5265 ), #4029, .F. ) ;
#18365=CARTESIAN_POINT ( 'NONE',  ( 5.000000000000007994, -56.56854249492410958, 56.56854249492351983 ) ) ;
#18413=CARTESIAN_POINT ( 'NONE',  ( 53.01450034489953111, 15.47727011842658307, 0.8544031610831416268 ) ) ;
#18420=CARTESIAN_POINT ( 'NONE',  ( 7.999999999999996447, 1.469527624586858429E-15, -1.540743955509788245E-31 ) ) ;
#18422=CARTESIAN_POINT ( 'NONE',  ( 47.98575327796820744, 15.47722964620001385, -0.8550501376822413624 ) ) ;
#18474=CARTESIAN_POINT ( 'NONE',  ( 49.32574372153255382, 15.31603864467538934, 2.381899414255259639 ) ) ;
#18538=DIRECTION ( 'NONE',  ( 1.000000000000000000, 1.836909530733573776E-16, -1.925929944387235853E-32 ) ) ;
#18677=DIRECTION ( 'NONE',  ( 0.000000000000000000, 0.7071067811865500152, -0.7071067811865449082 ) ) ;
#18683=DIRECTION ( 'NONE',  ( -1.000000000000000000, -1.836909530733573776E-16, 2.465190328815655050E-32 ) ) ;
#18722=CARTESIAN_POINT ( 'NONE',  ( 51.82989359177101107, 15.32891900549394038, 2.298613371999423727 ) ) ;
#18753=EDGE_CURVE ( 'NONE', #18771, #44393, #32809, .T. ) ;
#18771=VERTEX_POINT ( 'NONE', #6405 ) ;
#18795=CARTESIAN_POINT ( 'NONE',  ( 48.20074816270739859, 15.44360797527890483, 1.328834602619866967 ) ) ;
#18801=ADVANCED_FACE ( 'NONE', ( #1113 ), #43772, .F. ) ;
#18879=VECTOR ( 'NONE', #30536, 1000.000000000000000 ) ;
#18937=CARTESIAN_POINT ( 'NONE',  ( 43.00000000000000000, 0.000000000000000000, 12.50000000000000000 ) ) ;
#18956=ORIENTED_EDGE ( 'NONE', *, *, #1646, .T. ) ;
#19022=ORIENTED_EDGE ( 'NONE', *, *, #56510, .T. ) ;
#19024=DIRECTION ( 'NONE',  ( -1.000000000000000000, -3.673819061467147552E-16, 1.925929944387235306E-32 ) ) ;
#19053=CARTESIAN_POINT ( 'NONE',  ( 48.19985924247141185, 15.44373933981895952, -1.327350711001176631 ) ) ;
#19155=VECTOR ( 'NONE', #46233, 1000.000000000000000 ) ;
#19227=EDGE_LOOP ( 'NONE', ( #23087, #47498, #19022, #27535, #28345, #56112, #14577 ) ) ;
#19236=VECTOR ( 'NONE', #8691, 1000.000000000000000 ) ;
#19240=ORIENTED_EDGE ( 'NONE', *, *, #25179, .F. ) ;
#19260=EDGE_CURVE ( 'NONE', #61948, #28137, #51354, .T. ) ;
#19370=FACE_BOUND ( 'NONE', #25814, .T. ) ;
#19390=CARTESIAN_POINT ( 'NONE',  ( 43.00000000000000000, 5.682605120120046040E-15, -2.995852231480065614E-16 ) ) ;
#19409=AXIS2_PLACEMENT_3D ( 'NONE', #36142, #50823, #12952 ) ;
#19660=CARTESIAN_POINT ( 'NONE',  ( 47.85000000000000853, 15.50000000000000711, 1.598617397282144235E-15 ) ) ;
#19683=DIRECTION ( 'NONE',  ( 1.000000000000000000, 1.836909530733573776E-16, -1.925929944387235853E-32 ) ) ;
#19816=DIRECTION ( 'NONE',  ( 0.000000000000000000, 0.7071067811865421326, 0.7071067811865527908 ) ) ;
#19848=DIRECTION ( 'NONE',  ( 0.000000000000000000, -0.7071067811865435759, -0.7071067811865514585 ) ) ;
#19877=CIRCLE ( 'NONE', #57848, 2.649999999999992806 ) ;
#19878=CARTESIAN_POINT ( 'NONE',  ( 5.000000000000007994, -58.44237546506844438, 54.69470952477915660 ) ) ;
#19920=DIRECTION ( 'NONE',  ( 0.000000000000000000, 0.000000000000000000, 1.000000000000000000 ) ) ;
#19944=CARTESIAN_POINT ( 'NONE',  ( 5.000000000000007994, -58.44237546506844438, 54.69470952477916370 ) ) ;
#20057=DIRECTION ( 'NONE',  ( 1.000000000000000000, 1.836909530733573776E-16, -1.925929944387235853E-32 ) ) ;
#20149=CARTESIAN_POINT ( 'NONE',  ( 48.39340508532479390, 12.39581920280924088, 1.616942749076695662 ) ) ;
#20254=CARTESIAN_POINT ( 'NONE',  ( 5.000000000000007994, -56.56854249492331377, -56.56854249492430142 ) ) ;
#20376=EDGE_CURVE ( 'NONE', #59796, #61948, #44498, .T. ) ;
#20436=CIRCLE ( 'NONE', #55436, 2.649999999999999467 ) ;
#20457=VERTEX_POINT ( 'NONE', #58063 ) ;
#20507=CARTESIAN_POINT ( 'NONE',  ( 4.999999999999984901, 72.00000000000002842, -4.333342374871278042E-31 ) ) ;
#20534=DIRECTION ( 'NONE',  ( -1.000000000000000000, -1.836909530733580185E-16, 1.836909530733574022E-16 ) ) ;
#20583=EDGE_CURVE ( 'NONE', #32701, #1858, #12040, .T. ) ;
#20701=CARTESIAN_POINT ( 'NONE',  ( 50.50000000000000000, 12.21587082446438011, -2.649999999999992806 ) ) ;
#20707=CIRCLE ( 'NONE', #689, 12.50000000000000000 ) ;
#20803=ORIENTED_EDGE ( 'NONE', *, *, #9358, .F. ) ;
#20946=FILL_AREA_STYLE ('',( #1818 ) ) ;
#21069=ADVANCED_FACE ( 'NONE', ( #522 ), #27813, .T. ) ;
#21154=DIRECTION ( 'NONE',  ( 3.273063162220399693E-16, -1.000000000000000000, -5.236901059552639509E-15 ) ) ;
#21205=DIRECTION ( 'NONE',  ( -1.000000000000000000, -1.836909530733573776E-16, 1.925929944387235579E-32 ) ) ;
#21209=EDGE_LOOP ( 'NONE', ( #61258, #35094 ) ) ;
#21221=EDGE_CURVE ( 'NONE', #43044, #23359, #39531, .T. ) ;
#21274=ADVANCED_FACE ( 'NONE', ( #51220, #26188 ), #22421, .F. ) ;
#21327=CIRCLE ( 'NONE', #22309, 2.649999999999985700 ) ;
#21374=CARTESIAN_POINT ( 'NONE',  ( 48.39231140143691334, 12.39600195714815456, -1.615626833367223236 ) ) ;
#21488=DIRECTION ( 'NONE',  ( 1.000000000000000000, 1.836909530733573776E-16, -1.925929944387235853E-32 ) ) ;
#21743=ADVANCED_FACE ( 'NONE', ( #23574 ), #46478, .F. ) ;
#21765=AXIS2_PLACEMENT_3D ( 'NONE', #39975, #44358, #1387 ) ;
#21809=CYLINDRICAL_SURFACE ( 'NONE', #8776, 72.00000000000002842 ) ;
#21810=ORIENTED_EDGE ( 'NONE', *, *, #18753, .F. ) ;
#21854=EDGE_CURVE ( 'NONE', #31453, #1858, #47320, .T. ) ;
#21876=SURFACE_SIDE_STYLE ('',( #3663 ) ) ;
#21935=CARTESIAN_POINT ( 'NONE',  ( 7.999999999999983125, 80.00000000000001421, -9.340760230278089508E-32 ) ) ;
#21968=B_SPLINE_CURVE_WITH_KNOTS ( 'NONE', 3,
 ( #35179, #39576, #1939, #40207, #53022, #10122, #38963, #24521, #20149, #15757, #48335, #58316, #15444, #34553, #25137, #44279, #41127, #35800, #50487, #21374, #54865, #50186, #32016, #45208, #36115, #8185, #22302, #2558 ),
 .UNSPECIFIED., .F., .F.,
 ( 4, 2, 2, 2, 2, 2, 2, 2, 2, 2, 2, 2, 2, 4 ),
 ( 0.008308694440061006881, 0.009347008373300980805, 0.009866165339920957358, 0.01038532230654093391, 0.01090447927316091220, 0.01142363623978088875, 0.01246195017302085400, 0.01298110713964083576, 0.01350026410626081752, 0.01401942107288079928, 0.01453857803950078104, 0.01557689197274074455, 0.01609604893936073672, 0.01661520590598072888 ),
 .UNSPECIFIED. ) ;
#22022=ADVANCED_FACE ( 'NONE', ( #40479 ), #35462, .F. ) ;
#22053=CIRCLE ( 'NONE', #23046, 2.649999999999985700 ) ;
#22095=VERTEX_POINT ( 'NONE', #37949 ) ;
#22127=ADVANCED_FACE ( 'NONE', ( #18198 ), #60463, .F. ) ;
#22211=CARTESIAN_POINT ( 'NONE',  ( 4.999999999999997335, -2.784000523420839360E-13, 80.00000000000001421 ) ) ;
#22251=VERTEX_POINT ( 'NONE', #47939 ) ;
#22302=CARTESIAN_POINT ( 'NONE',  ( 50.32441585594579436, 12.21587082446438011, -2.649999999999992806 ) ) ;
#22309=AXIS2_PLACEMENT_3D ( 'NONE', #57527, #52853, #5527 ) ;
#22317=CARTESIAN_POINT ( 'NONE',  ( 4.999999999999983125, 80.00000000000001421, -3.562970397116383044E-32 ) ) ;
#22400=CYLINDRICAL_SURFACE ( 'NONE', #2380, 2.649999999999992806 ) ;
#22421=PLANE ( 'NONE',  #41538 ) ;
#22481=DIRECTION ( 'NONE',  ( -1.000000000000000000, -0.000000000000000000, 1.925929944387235853E-32 ) ) ;
#22496=CARTESIAN_POINT ( 'NONE',  ( 4.999999999999984901, 72.00000000000002842, -9.629649721936170507E-32 ) ) ;
#22564=DIRECTION ( 'NONE',  ( -1.000000000000000000, -1.836909530733573776E-16, 1.925929944387235853E-32 ) ) ;
#22596=VERTEX_POINT ( 'NONE', #59319 ) ;
#22645=DIRECTION ( 'NONE',  ( -1.000000000000000000, -1.836909530733573776E-16, 1.925929944387235579E-32 ) ) ;
#22657=CARTESIAN_POINT ( 'NONE',  ( 58.00000000000000000, 8.437969416220405915E-15, -2.995852231480068572E-16 ) ) ;
#22679=ORIENTED_EDGE ( 'NONE', *, *, #40986, .F. ) ;
#22777=DIRECTION ( 'NONE',  ( 0.000000000000000000, 0.000000000000000000, -1.000000000000000000 ) ) ;
#22815=DIRECTION ( 'NONE',  ( 0.000000000000000000, 0.000000000000000000, -1.000000000000000000 ) ) ;
#22822=AXIS2_PLACEMENT_3D ( 'NONE', #42222, #19024, #22777 ) ;
#22838=EDGE_CURVE ( 'NONE', #44393, #18771, #2939, .T. ) ;
#22842=CIRCLE ( 'NONE', #23824, 2.649999999999997691 ) ;
#22865=CARTESIAN_POINT ( 'NONE',  ( 49.81163791968438659, 15.28633307723669077, 2.564998524509804145 ) ) ;
#22869=EDGE_CURVE ( 'NONE', #24288, #26981, #4906, .T. ) ;
#22871=MECHANICAL_DESIGN_GEOMETRIC_PRESENTATION_REPRESENTATION('',(#49872),#60856);
#22880=DIRECTION ( 'NONE',  ( 0.000000000000000000, 3.491481338843138088E-15, -1.000000000000000000 ) ) ;
#22995=EDGE_CURVE ( 'NONE', #1858, #31453, #6906, .T. ) ;
#23041=CARTESIAN_POINT ( 'NONE',  ( 58.00000000000000000, 8.437969416220405915E-15, -2.995852231480068572E-16 ) ) ;
#23046=AXIS2_PLACEMENT_3D ( 'NONE', #3435, #37299, #22880 ) ;
#23059=DIRECTION ( 'NONE',  ( 0.000000000000000000, -0.7071067811865449082, -0.7071067811865500152 ) ) ;
#23087=ORIENTED_EDGE ( 'NONE', *, *, #1646, .F. ) ;
#23266=EDGE_CURVE ( 'NONE', #25227, #59695, #57569, .T. ) ;
#23359=VERTEX_POINT ( 'NONE', #50055 ) ;
#23419=DIRECTION ( 'NONE',  ( 1.836766033387207149E-16, -1.000000000000000000, 0.000000000000000000 ) ) ;
#23422=CIRCLE ( 'NONE', #12428, 85.00000000000001421 ) ;
#23468=VECTOR ( 'NONE', #61492, 1000.000000000000000 ) ;
#23574=FACE_OUTER_BOUND ( 'NONE', #46921, .T. ) ;
#23641=CARTESIAN_POINT ( 'NONE',  ( 4.999999999999986677, 54.69470952477936976, 58.44237546506825964 ) ) ;
#23665=SURFACE_SIDE_STYLE ('',( #46878 ) ) ;
#23729=DIRECTION ( 'NONE',  ( -1.000000000000000000, -1.836909530733573776E-16, 1.925929944387235579E-32 ) ) ;
#23730=CARTESIAN_POINT ( 'NONE',  ( 47.93459374525478722, 15.48572582901846140, -0.6863552170468703029 ) ) ;
#23824=AXIS2_PLACEMENT_3D ( 'NONE', #37484, #61857, #38114 ) ;
#23828=DIRECTION ( 'NONE',  ( -1.000000000000000000, -1.836909530733573776E-16, 1.925929944387235853E-32 ) ) ;
#23850=DIRECTION ( 'NONE',  ( -1.000000000000000000, -1.836909530733573776E-16, 2.465190328815682145E-32 ) ) ;
#23854=LINE ( 'NONE', #38285, #50293 ) ;
#23859=EDGE_LOOP ( 'NONE', ( #25749, #26790 ) ) ;
#23924=CARTESIAN_POINT ( 'NONE',  ( 4.999999999999983125, 80.00000000000001421, -2.649999999999992806 ) ) ;
#24027=CARTESIAN_POINT ( 'NONE',  ( 53.14999999999999147, 15.50000000000000711, 0.1731622330692809963 ) ) ;
#24061=CARTESIAN_POINT ( 'NONE',  ( 53.06512528815419927, 15.48567863024351432, -0.6878158681035048128 ) ) ;
#24251=LINE ( 'NONE', #38688, #60610 ) ;
#24288=VERTEX_POINT ( 'NONE', #28405 ) ;
#24330=CARTESIAN_POINT ( 'NONE',  ( 58.00000000000000000, -15.49999999999999112, -2.995852231480067093E-16 ) ) ;
#24346=CARTESIAN_POINT ( 'NONE',  ( 48.86911069238522742, 15.35671945348452638, -2.116951128576620711 ) ) ;
#24389=EDGE_LOOP ( 'NONE', ( #13136, #39410 ) ) ;
#24513=AXIS2_PLACEMENT_3D ( 'NONE', #14969, #5523, #34079 ) ;
#24521=CARTESIAN_POINT ( 'NONE',  ( 48.50503732531682033, 12.37710729184128944, 1.752842796636026490 ) ) ;
#24544=EDGE_LOOP ( 'NONE', ( #9962, #30973 ) ) ;
#24830=CARTESIAN_POINT ( 'NONE',  ( 4.999999999999996447, 2.649999999999714362, 80.00000000000002842 ) ) ;
#24880=DIRECTION ( 'NONE',  ( 0.000000000000000000, 0.000000000000000000, 1.000000000000000000 ) ) ;
#24894=ORIENTED_EDGE ( 'NONE', *, *, #20583, .F. ) ;
#24916=CARTESIAN_POINT ( 'NONE',  ( 5.000000000000012434, -80.00000000000001421, -1.569632904675596344E-31 ) ) ;
#24969=AXIS2_PLACEMENT_3D ( 'NONE', #57637, #323, #958 ) ;
#25084=CARTESIAN_POINT ( 'NONE',  ( 52.11715515643994223, 12.32162532810768241, 2.106428410961948217 ) ) ;
#25100=CARTESIAN_POINT ( 'NONE',  ( 7.999999999999996447, 1.469527624586858429E-15, -1.540743955509788245E-31 ) ) ;
#25115=DIRECTION ( 'NONE',  ( 0.000000000000000000, 0.7071067811865382469, 0.7071067811865566766 ) ) ;
#25137=CARTESIAN_POINT ( 'NONE',  ( 47.86699140808116937, 12.49636532218518425, -0.3460709571827094710 ) ) ;
#25179=EDGE_CURVE ( 'NONE', #12452, #57986, #22053, .T. ) ;
#25227=VERTEX_POINT ( 'NONE', #8771 ) ;
#25236=EDGE_CURVE ( 'NONE', #40875, #29142, #32077, .T. ) ;
#25282=ORIENTED_EDGE ( 'NONE', *, *, #3459, .F. ) ;
#25292=STYLED_ITEM ( 'NONE', ( #60309 ), #31769 ) ;
#25356=CARTESIAN_POINT ( 'NONE',  ( 58.00000000000000000, 8.437969416220405915E-15, -2.995852231480068572E-16 ) ) ;
#25371=ORIENTED_EDGE ( 'NONE', *, *, #60027, .F. ) ;
#25394=FACE_OUTER_BOUND ( 'NONE', #14309, .T. ) ;
#25419=PLANE ( 'NONE',  #33730 ) ;
#25443=VERTEX_POINT ( 'NONE', #49682 ) ;
#25509=CIRCLE ( 'NONE', #43529, 2.649999999999992806 ) ;
#25526=FACE_OUTER_BOUND ( 'NONE', #702, .T. ) ;
#25583=ORIENTED_EDGE ( 'NONE', *, *, #17947, .F. ) ;
#25600=CARTESIAN_POINT ( 'NONE',  ( 4.999999999999983125, 80.00000000000001421, 2.649999999999999467 ) ) ;
#25658=EDGE_LOOP ( 'NONE', ( #57363, #14198 ) ) ;
#25733=DIRECTION ( 'NONE',  ( -1.000000000000000000, -1.836909530733554547E-16, -1.836909530733573529E-16 ) ) ;
#25749=ORIENTED_EDGE ( 'NONE', *, *, #20376, .F. ) ;
#25814=EDGE_LOOP ( 'NONE', ( #34035, #9295 ) ) ;
#25827=CIRCLE ( 'NONE', #43889, 2.649999999999999467 ) ;
#25840=DIRECTION ( 'NONE',  ( 3.273063162220399693E-16, -1.000000000000000000, -5.236901059552639509E-15 ) ) ;
#25853=COLOUR_RGB ( '', 0.66274510, 0.83137255, 0.94901961) ;
#25877=AXIS2_PLACEMENT_3D ( 'NONE', #4130, #37697, #42096 ) ;
#25989=DIRECTION ( 'NONE',  ( 0.000000000000000000, 0.000000000000000000, 1.000000000000000000 ) ) ;
#25999=EDGE_LOOP ( 'NONE', ( #20803, #59336, #49265, #8232 ) ) ;
#26018=CARTESIAN_POINT ( 'NONE',  ( 52.25045007007695830, 12.34004751916969411, 1.997177200709687739 ) ) ;
#26048=ORIENTED_EDGE ( 'NONE', *, *, #21854, .F. ) ;
#26052=ORIENTED_EDGE ( 'NONE', *, *, #61843, .T. ) ;
#26102=FACE_OUTER_BOUND ( 'NONE', #50303, .T. ) ;
#26122=UNCERTAINTY_MEASURE_WITH_UNIT (LENGTH_MEASURE( 1.000000000000000082E-05 ), #60994, 'distance_accuracy_value', 'NONE');
#26136=DIRECTION ( 'NONE',  ( -1.000000000000000000, -0.000000000000000000, -0.000000000000000000 ) ) ;
#26157=CARTESIAN_POINT ( 'NONE',  ( 4.999999999999997335, -2.784000523420839360E-13, 80.00000000000001421 ) ) ;
#26188=FACE_OUTER_BOUND ( 'NONE', #9222, .T. ) ;
#26256=CARTESIAN_POINT ( 'NONE',  ( 8.000000000000007105, -56.56854249492410958, 56.56854249492351983 ) ) ;
#26297=AXIS2_PLACEMENT_3D ( 'NONE', #15418, #34531, #25115 ) ;
#26447=FACE_BOUND ( 'NONE', #43513, .T. ) ;
#26502=CIRCLE ( 'NONE', #16496, 2.649999999999985700 ) ;
#26557=CARTESIAN_POINT ( 'NONE',  ( 4.999999999999986677, 58.44237546506807490, 54.69470952477956871 ) ) ;
#26701=VERTEX_POINT ( 'NONE', #15462 ) ;
#26790=ORIENTED_EDGE ( 'NONE', *, *, #12608, .F. ) ;
#26933=CARTESIAN_POINT ( 'NONE',  ( 5.000000000000012434, -80.00000000000001421, -1.569632904675596344E-31 ) ) ;
#26941=DIRECTION ( 'NONE',  ( 0.000000000000000000, -1.000000000000000000, 0.000000000000000000 ) ) ;
#26953=CIRCLE ( 'NONE', #58948, 15.50000000000000000 ) ;
#26958=CARTESIAN_POINT ( 'NONE',  ( 40.00000000000000000, 1.530808498934191521E-15, -12.50000000000000000 ) ) ;
#26981=VERTEX_POINT ( 'NONE', #26557 ) ;
#27107=B_SPLINE_CURVE_WITH_KNOTS ( 'NONE', 3,
 ( #19660, #42246, #37860, #23730, #18422, #42860, #19053, #47858, #61912, #24346, #43477, #52847, #56921, #9625, #9314, #38780 ),
 .UNSPECIFIED., .F., .F.,
 ( 4, 2, 2, 2, 2, 2, 2, 4 ),
 ( 0.01245102954896282026, 0.01296947782926336466, 0.01348792610956391080, 0.01400637438986445521, 0.01452482267016500135, 0.01556171923076610578, 0.01608016751106664671, 0.01659861579136719112 ),
 .UNSPECIFIED. ) ;
#27122=EDGE_LOOP ( 'NONE', ( #4151, #16182, #60857, #42289 ) ) ;
#27207=ORIENTED_EDGE ( 'NONE', *, *, #56510, .F. ) ;
#27429=FILL_AREA_STYLE_COLOUR ( '', #274 ) ;
#27437=VECTOR ( 'NONE', #42434, 1000.000000000000000 ) ;
#27492=LINE ( 'NONE', #11887, #1810 ) ;
#27498=AXIS2_PLACEMENT_3D ( 'NONE', #3253, #55885, #13009 ) ;
#27535=ORIENTED_EDGE ( 'NONE', *, *, #48508, .T. ) ;
#27565=ORIENTED_EDGE ( 'NONE', *, *, #23266, .F. ) ;
#27667=EDGE_LOOP ( 'NONE', ( #7248, #38654, #36956, #48403 ) ) ;
#27683=FACE_BOUND ( 'NONE', #23859, .T. ) ;
#27688=ORIENTED_EDGE ( 'NONE', *, *, #3868, .T. ) ;
#27801=CARTESIAN_POINT ( 'NONE',  ( 50.84889841487235174, 15.27482646519414367, 2.632653459949275465 ) ) ;
#27813=CYLINDRICAL_SURFACE ( 'NONE', #51513, 15.50000000000000000 ) ;
#27822=CARTESIAN_POINT ( 'NONE',  ( 43.00000000000000000, 0.000000000000000000, 0.000000000000000000 ) ) ;
#27831=ORIENTED_EDGE ( 'NONE', *, *, #39069, .T. ) ;
#27980=DIRECTION ( 'NONE',  ( -1.000000000000000000, -1.836909530733573776E-16, 1.925929944387235853E-32 ) ) ;
#28038=LINE ( 'NONE', #23641, #19155 ) ;
#28062=CARTESIAN_POINT ( 'NONE',  ( 4.999999999999997335, 9.184547653667864935E-16, -9.629649721936170507E-32 ) ) ;
#28079=CIRCLE ( 'NONE', #58061, 15.50000000000000000 ) ;
#28082=EDGE_CURVE ( 'NONE', #14994, #12923, #40166, .T. ) ;
#28109=CARTESIAN_POINT ( 'NONE',  ( 51.67479428703781963, 15.31607246706614056, 2.381689993923809201 ) ) ;
#28126=EDGE_LOOP ( 'NONE', ( #3162, #13095 ) ) ;
#28137=VERTEX_POINT ( 'NONE', #26958 ) ;
#28138=FACE_BOUND ( 'NONE', #28275, .T. ) ;
#28153=VERTEX_POINT ( 'NONE', #2514 ) ;
#28161=ORIENTED_EDGE ( 'NONE', *, *, #9848, .T. ) ;
#28199=EDGE_CURVE ( 'NONE', #30745, #37740, #33874, .T. ) ;
#28217=FACE_OUTER_BOUND ( 'NONE', #5933, .T. ) ;
#28275=EDGE_LOOP ( 'NONE', ( #55890, #27831 ) ) ;
#28345=ORIENTED_EDGE ( 'NONE', *, *, #9339, .T. ) ;
#28405=CARTESIAN_POINT ( 'NONE',  ( 4.999999999999986677, 54.69470952477936976, 58.44237546506825964 ) ) ;
#28433=DIRECTION ( 'NONE',  ( 1.000000000000000000, 1.836909530733573776E-16, -1.925929944387235853E-32 ) ) ;
#28436=CARTESIAN_POINT ( 'NONE',  ( 50.50000000000000000, 15.27178771460631168, -2.649999999999992806 ) ) ;
#28441=CARTESIAN_POINT ( 'NONE',  ( 50.50000000000000000, 15.27178771460631168, 2.649999999999992806 ) ) ;
#28488=EDGE_CURVE ( 'NONE', #243, #8457, #19877, .T. ) ;
#28561=VECTOR ( 'NONE', #52414, 1000.000000000000000 ) ;
#28697=AXIS2_PLACEMENT_3D ( 'NONE', #26933, #2488, #36046 ) ;
#28867=CIRCLE ( 'NONE', #41917, 2.649999999999997691 ) ;
#28883=DIRECTION ( 'NONE',  ( -1.000000000000000000, -1.836909530733573776E-16, -1.361838123766432833E-32 ) ) ;
#28919=DIRECTION ( 'NONE',  ( -1.000000000000000000, -1.836909530733573776E-16, 2.465190328815682145E-32 ) ) ;
#28967=CIRCLE ( 'NONE', #17982, 2.649999999999999467 ) ;
#28974=CARTESIAN_POINT ( 'NONE',  ( 4.999999999999998224, -2.649999999999153921, -80.00000000000004263 ) ) ;
#29014=CARTESIAN_POINT ( 'NONE',  ( 50.50000000000000000, 0.000000000000000000, 2.649999999999992806 ) ) ;
#29047=LINE ( 'NONE', #48159, #34526 ) ;
#29067=CARTESIAN_POINT ( 'NONE',  ( 52.11657354882707693, 15.35644106150795807, -2.106932783932539799 ) ) ;
#29142=VERTEX_POINT ( 'NONE', #14639 ) ;
#29297=CARTESIAN_POINT ( 'NONE',  ( 7.999999999999986677, 56.56854249492450037, -56.56854249492312192 ) ) ;
#29451=VECTOR ( 'NONE', #20534, 1000.000000000000000 ) ;
#29507=VERTEX_POINT ( 'NONE', #19878 ) ;
#29514=ORIENTED_EDGE ( 'NONE', *, *, #39380, .F. ) ;
#29671=DIRECTION ( 'NONE',  ( -1.000000000000000000, -3.135800716341471541E-16, -1.298891185607920445E-16 ) ) ;
#29738=LINE ( 'NONE', #44494, #49972 ) ;
#29764=AXIS2_PLACEMENT_3D ( 'NONE', #4633, #4957, #48502 ) ;
#29773=VERTEX_POINT ( 'NONE', #9145 ) ;
#29783=CARTESIAN_POINT ( 'NONE',  ( 50.67563028805193426, 12.21587082446438011, -2.649999999999992362 ) ) ;
#29877=PRODUCT_DEFINITION_FORMATION_WITH_SPECIFIED_SOURCE ( 'ANY', '', #7765, .NOT_KNOWN. ) ;
#29907=ORIENTED_EDGE ( 'NONE', *, *, #47607, .T. ) ;
#29972=ORIENTED_EDGE ( 'NONE', *, *, #47607, .F. ) ;
#30276=EDGE_CURVE ( 'NONE', #243, #13900, #40706, .T. ) ;
#30295=ORIENTED_EDGE ( 'NONE', *, *, #59760, .F. ) ;
#30389=CARTESIAN_POINT ( 'NONE',  ( 53.15006792977867178, 12.50001440111202022, 0.1723589083839783265 ) ) ;
#30404=EDGE_CURVE ( 'NONE', #58558, #18771, #13415, .T. ) ;
#30525=CARTESIAN_POINT ( 'NONE',  ( 4.999999999999998224, -2.650000000000271250, 80.00000000000000000 ) ) ;
#30535=ORIENTED_EDGE ( 'NONE', *, *, #32108, .T. ) ;
#30536=DIRECTION ( 'NONE',  ( -1.000000000000000000, -3.135800716341489291E-16, 1.298891185607901956E-16 ) ) ;
#30544=DIRECTION ( 'NONE',  ( 0.000000000000000000, 0.000000000000000000, 1.000000000000000000 ) ) ;
#30568=CIRCLE ( 'NONE', #33588, 72.00000000000002842 ) ;
#30703=CARTESIAN_POINT ( 'NONE',  ( 52.11660573588833500, 12.32154690648379436, -2.106899540995512687 ) ) ;
#30745=VERTEX_POINT ( 'NONE', #57361 ) ;
#30806=ORIENTED_EDGE ( 'NONE', *, *, #51597, .T. ) ;
#30807=ORIENTED_EDGE ( 'NONE', *, *, #56910, .F. ) ;
#30915=FACE_BOUND ( 'NONE', #55013, .T. ) ;
#30933=VECTOR ( 'NONE', #31334, 1000.000000000000000 ) ;
#30973=ORIENTED_EDGE ( 'NONE', *, *, #3459, .T. ) ;
#30985=DIRECTION ( 'NONE',  ( 0.000000000000000000, 0.000000000000000000, -1.000000000000000000 ) ) ;
#31102=DIRECTION ( 'NONE',  ( 0.000000000000000000, 0.000000000000000000, -1.000000000000000000 ) ) ;
#31111=DIRECTION ( 'NONE',  ( -1.000000000000000000, -5.380183451256670742E-17, 1.298891185607911324E-16 ) ) ;
#31143=CARTESIAN_POINT ( 'NONE',  ( 8.000000000000000000, 0.000000000000000000, 0.000000000000000000 ) ) ;
#31274=DIRECTION ( 'NONE',  ( 0.000000000000000000, 0.7071067811865500152, -0.7071067811865449082 ) ) ;
#31333=ORIENTED_EDGE ( 'NONE', *, *, #19260, .T. ) ;
#31334=DIRECTION ( 'NONE',  ( 1.000000000000000000, 1.836909530733573776E-16, -1.925929944387235853E-32 ) ) ;
#31453=VERTEX_POINT ( 'NONE', #10568 ) ;
#31544=EDGE_CURVE ( 'NONE', #96, #15197, #21327, .T. ) ;
#31564=CIRCLE ( 'NONE', #50547, 75.00000000000001421 ) ;
#31603=ORIENTED_EDGE ( 'NONE', *, *, #1079, .T. ) ;
#31641=EDGE_LOOP ( 'NONE', ( #37032, #45109, #33306, #56672 ) ) ;
#31658=CIRCLE ( 'NONE', #8609, 2.649999999999992806 ) ;
#31769=MANIFOLD_SOLID_BREP ( 'M5 Clearance Hole2', #11054 ) ;
#31791=LINE ( 'NONE', #56498, #60651 ) ;
#31840=AXIS2_PLACEMENT_3D ( 'NONE', #46022, #46316, #50076 ) ;
#31859=ORIENTED_EDGE ( 'NONE', *, *, #11831, .T. ) ;
#31865=ORIENTED_EDGE ( 'NONE', *, *, #30404, .T. ) ;
#31931=ORIENTED_EDGE ( 'NONE', *, *, #60677, .T. ) ;
#31942=AXIS2_PLACEMENT_3D ( 'NONE', #2499, #59826, #16303 ) ;
#32016=CARTESIAN_POINT ( 'NONE',  ( 49.16300155221411217, 12.28471438860442078, -2.313890179308903505 ) ) ;
#32018=CARTESIAN_POINT ( 'NONE',  ( 4.999999999999997335, 8.388739760877188892E-13, -80.00000000000001421 ) ) ;
#32027=CARTESIAN_POINT ( 'NONE',  ( 5.000000000000007994, -56.56854249492410958, 56.56854249492351983 ) ) ;
#32035=ORIENTED_EDGE ( 'NONE', *, *, #28488, .F. ) ;
#32077=CIRCLE ( 'NONE', #56016, 15.50000000000000000 ) ;
#32085=FACE_OUTER_BOUND ( 'NONE', #55916, .T. ) ;
#32108=EDGE_CURVE ( 'NONE', #33073, #4875, #5329, .T. ) ;
#32157=ORIENTED_EDGE ( 'NONE', *, *, #45187, .T. ) ;
#32219=CARTESIAN_POINT ( 'NONE',  ( 7.999999999999983125, 80.00000000000001421, -2.649999999999992806 ) ) ;
#32236=CYLINDRICAL_SURFACE ( 'NONE', #13477, 2.649999999999992806 ) ;
#32274=CARTESIAN_POINT ( 'NONE',  ( 43.00000000000000000, 1.530808498934191521E-15, -12.50000000000000000 ) ) ;
#32337=DIRECTION ( 'NONE',  ( -1.000000000000000000, -0.000000000000000000, 1.925929944387235853E-32 ) ) ;
#32379=CARTESIAN_POINT ( 'NONE',  ( 40.00000000000000000, 7.347638122934295104E-15, -7.703719777548943412E-31 ) ) ;
#32643=ORIENTED_EDGE ( 'NONE', *, *, #8861, .T. ) ;
#32701=VERTEX_POINT ( 'NONE', #54113 ) ;
#32809=CIRCLE ( 'NONE', #56782, 72.00000000000002842 ) ;
#32841=DIRECTION ( 'NONE',  ( -1.000000000000000000, -5.380183451256491399E-17, -1.298891185607892835E-16 ) ) ;
#32897=CARTESIAN_POINT ( 'NONE',  ( 48.88223999046894619, 15.35656115023722812, 2.106076572069662589 ) ) ;
#32959=DIRECTION ( 'NONE',  ( 0.000000000000000000, -1.047444401652941269E-14, 1.000000000000000000 ) ) ;
#33073=VERTEX_POINT ( 'NONE', #2661 ) ;
#33099=DIRECTION ( 'NONE',  ( 0.000000000000000000, 3.491481338843138088E-15, -1.000000000000000000 ) ) ;
#33207=ADVANCED_FACE ( 'NONE', ( #59990 ), #22400, .F. ) ;
#33241=DIRECTION ( 'NONE',  ( 1.836909530733573776E-16, -1.000000000000000000, 0.000000000000000000 ) ) ;
#33255=ORIENTED_EDGE ( 'NONE', *, *, #39405, .F. ) ;
#33306=ORIENTED_EDGE ( 'NONE', *, *, #43181, .T. ) ;
#33324=EDGE_CURVE ( 'NONE', #37740, #9990, #6335, .T. ) ;
#33396=EDGE_CURVE ( 'NONE', #37740, #30745, #36450, .T. ) ;
#33406=AXIS2_PLACEMENT_3D ( 'NONE', #58351, #58662, #39928 ) ;
#33452=ORIENTED_EDGE ( 'NONE', *, *, #43108, .F. ) ;
#33457=DIRECTION ( 'NONE',  ( 0.000000000000000000, -1.000000000000000000, 0.000000000000000000 ) ) ;
#33471=ADVANCED_FACE ( 'NONE', ( #60833 ), #56135, .F. ) ;
#33476=FACE_BOUND ( 'NONE', #28126, .T. ) ;
#33588=AXIS2_PLACEMENT_3D ( 'NONE', #28062, #14290, #19920 ) ;
#33618=ORIENTED_EDGE ( 'NONE', *, *, #61572, .T. ) ;
#33633=ORIENTED_EDGE ( 'NONE', *, *, #20376, .T. ) ;
#33730=AXIS2_PLACEMENT_3D ( 'NONE', #17278, #44565, #58931 ) ;
#33787=CARTESIAN_POINT ( 'NONE',  ( 50.84796438615735781, 15.27481071999428508, -2.632742199681755491 ) ) ;
#33790=FACE_BOUND ( 'NONE', #3377, .T. ) ;
#33800=EDGE_CURVE ( 'NONE', #4875, #33073, #23422, .T. ) ;
#33874=CIRCLE ( 'NONE', #60848, 2.649999999999985700 ) ;
#33939=ORIENTED_EDGE ( 'NONE', *, *, #36302, .F. ) ;
#34015=CARTESIAN_POINT ( 'NONE',  ( 5.000000000000007994, -58.44237546506768410, -54.69470952477996661 ) ) ;
#34035=ORIENTED_EDGE ( 'NONE', *, *, #28199, .T. ) ;
#34043=LINE ( 'NONE', #19944, #18879 ) ;
#34053=EDGE_LOOP ( 'NONE', ( #55421, #30535, #18270, #25282 ) ) ;
#34065=ADVANCED_BREP_SHAPE_REPRESENTATION ( '', ( #31769, #14677 ), #14881 ) ;
#34079=DIRECTION ( 'NONE',  ( 3.273063162220391312E-16, -1.000000000000000000, -5.236901059552626099E-15 ) ) ;
#34132=CARTESIAN_POINT ( 'NONE',  ( 47.98582422161447880, 15.47721683621552202, 0.8553894437622007185 ) ) ;
#34434=CARTESIAN_POINT ( 'NONE',  ( 47.85000000000000853, 15.50000000000000711, 1.598617397282144235E-15 ) ) ;
#34439=CARTESIAN_POINT ( 'NONE',  ( 4.999999999999986677, 58.44237546506882808, -54.69470952477875159 ) ) ;
#34526=VECTOR ( 'NONE', #32841, 1000.000000000000000 ) ;
#34531=DIRECTION ( 'NONE',  ( -1.000000000000000000, -5.380183451256491399E-17, -1.298891185607892835E-16 ) ) ;
#34553=CARTESIAN_POINT ( 'NONE',  ( 47.84992101484482419, 12.50001674485125669, -0.1737107653014904884 ) ) ;
#34658=AXIS2_PLACEMENT_3D ( 'NONE', #32018, #12004, #42053 ) ;
#34667=CARTESIAN_POINT ( 'NONE',  ( 43.00000000000000000, 0.000000000000000000, 0.000000000000000000 ) ) ;
#34720=CIRCLE ( 'NONE', #15718, 12.50000000000000000 ) ;
#34882=CIRCLE ( 'NONE', #25877, 85.00000000000001421 ) ;
#35058=CARTESIAN_POINT ( 'NONE',  ( 47.93486876061941615, 15.48568014845115748, 0.6873655611129172449 ) ) ;
#35094=ORIENTED_EDGE ( 'NONE', *, *, #21221, .F. ) ;
#35126=CARTESIAN_POINT ( 'NONE',  ( 52.81518117642549726, 12.43264790761136851, -1.334736769217753638 ) ) ;
#35179=CARTESIAN_POINT ( 'NONE',  ( 50.50000000000000000, 12.21587082446438011, 2.649999999999992806 ) ) ;
#35215=FACE_OUTER_BOUND ( 'NONE', #27667, .T. ) ;
#35244=DIRECTION ( 'NONE',  ( -1.000000000000000000, -3.673819061467147552E-16, 1.925929944387235306E-32 ) ) ;
#35366=ORIENTED_EDGE ( 'NONE', *, *, #3651, .T. ) ;
#35368=CARTESIAN_POINT ( 'NONE',  ( 47.86731964337302969, 15.49701252645352945, 0.3483731184818048554 ) ) ;
#35462=CYLINDRICAL_SURFACE ( 'NONE', #52306, 2.649999999999992806 ) ;
#35469=CARTESIAN_POINT ( 'NONE',  ( 7.999999999999983125, 80.00000000000001421, 2.649999999999992806 ) ) ;
#35618=AXIS2_PLACEMENT_3D ( 'NONE', #61439, #22645, #4729 ) ;
#35641=DIRECTION ( 'NONE',  ( 1.836909530733573776E-16, -1.000000000000000000, 0.000000000000000000 ) ) ;
#35655=AXIS2_PLACEMENT_3D ( 'NONE', #39113, #48476, #58780 ) ;
#35708=DIRECTION ( 'NONE',  ( -1.000000000000000000, -0.000000000000000000, -0.000000000000000000 ) ) ;
#35777=CARTESIAN_POINT ( 'NONE',  ( 8.000000000000012434, -85.00000000000001421, -1.540743955509788245E-31 ) ) ;
#35800=CARTESIAN_POINT ( 'NONE',  ( 48.11837490430890085, 12.44569835165631311, -1.174889345006233432 ) ) ;
#35913=CIRCLE ( 'NONE', #17887, 2.649999999999992806 ) ;
#36009=ORIENTED_EDGE ( 'NONE', *, *, #16131, .T. ) ;
#36046=DIRECTION ( 'NONE',  ( 0.000000000000000000, 0.000000000000000000, -1.000000000000000000 ) ) ;
#36115=CARTESIAN_POINT ( 'NONE',  ( 49.80929115161121956, 12.23419022400559442, -2.564334511966932517 ) ) ;
#36142=CARTESIAN_POINT ( 'NONE',  ( 5.000000000000012434, -80.00000000000001421, -1.569632904675596344E-31 ) ) ;
#36188=DIRECTION ( 'NONE',  ( -1.000000000000000000, -1.836909530733580185E-16, 1.836909530733574022E-16 ) ) ;
#36213=CARTESIAN_POINT ( 'NONE',  ( 50.50000000000000000, 0.000000000000000000, 0.000000000000000000 ) ) ;
#36241=ORIENTED_EDGE ( 'NONE', *, *, #6561, .F. ) ;
#36294=CARTESIAN_POINT ( 'NONE',  ( 4.999999999999982236, 85.00000000000001421, 1.040949779275250495E-14 ) ) ;
#36302=EDGE_CURVE ( 'NONE', #29142, #40875, #15657, .T. ) ;
#36421=CIRCLE ( 'NONE', #37403, 2.649999999999992806 ) ;
#36450=CIRCLE ( 'NONE', #33406, 2.649999999999985700 ) ;
#36643=VERTEX_POINT ( 'NONE', #51564 ) ;
#36732=CYLINDRICAL_SURFACE ( 'NONE', #34658, 2.649999999999992806 ) ;
#36916=DIRECTION ( 'NONE',  ( 0.000000000000000000, 0.000000000000000000, 1.000000000000000000 ) ) ;
#36921=PRESENTATION_STYLE_ASSIGNMENT (( #41015 ) ) ;
#36956=ORIENTED_EDGE ( 'NONE', *, *, #5129, .T. ) ;
#37032=ORIENTED_EDGE ( 'NONE', *, *, #30276, .F. ) ;
#37206=CARTESIAN_POINT ( 'NONE',  ( 5.000000000000012434, -80.00000000000001421, 2.649999999999999467 ) ) ;
#37299=DIRECTION ( 'NONE',  ( -1.000000000000000000, -1.836909530733573776E-16, 2.465190328815655050E-32 ) ) ;
#37368=EDGE_CURVE ( 'NONE', #13900, #29507, #46692, .T. ) ;
#37403=AXIS2_PLACEMENT_3D ( 'NONE', #40432, #15995, #49183 ) ;
#37408=VERTEX_POINT ( 'NONE', #58202 ) ;
#37437=VECTOR ( 'NONE', #15791, 1000.000000000000000 ) ;
#37479=DIRECTION ( 'NONE',  ( -1.000000000000000000, -1.836909530733573776E-16, 1.925929944387235853E-32 ) ) ;
#37484=CARTESIAN_POINT ( 'NONE',  ( 7.999999999999986677, 56.56854249492371878, 56.56854249492391062 ) ) ;
#37532=CARTESIAN_POINT ( 'NONE',  ( 52.88134325800242408, 15.45619532895059045, 1.175551374349551370 ) ) ;
#37562=CARTESIAN_POINT ( 'NONE',  ( 50.67548179587118540, 15.27178771460630813, -2.649999999999993694 ) ) ;
#37601=CARTESIAN_POINT ( 'NONE',  ( 50.50000000000000000, 15.27178771460631168, 2.649999999999992806 ) ) ;
#37669=CIRCLE ( 'NONE', #35655, 75.00000000000001421 ) ;
#37697=DIRECTION ( 'NONE',  ( -1.000000000000000000, -1.836909530733573776E-16, 1.925929944387235853E-32 ) ) ;
#37740=VERTEX_POINT ( 'NONE', #13023 ) ;
#37852=CARTESIAN_POINT ( 'NONE',  ( 50.50000000000000000, 15.27178771460631168, 2.649999999999992806 ) ) ;
#37860=CARTESIAN_POINT ( 'NONE',  ( 47.86716078833156729, 15.49703963710948784, -0.3472037173684915934 ) ) ;
#37862=DIRECTION ( 'NONE',  ( -1.000000000000000000, -1.836909530733573776E-16, 1.925929944387235853E-32 ) ) ;
#37921=CARTESIAN_POINT ( 'NONE',  ( 48.11924514954072407, 15.45610412777417686, 1.176765604160352252 ) ) ;
#37949=CARTESIAN_POINT ( 'NONE',  ( 43.00000000000000000, 9.184850993605153466E-15, -75.00000000000001421 ) ) ;
#37960=FACE_BOUND ( 'NONE', #5062, .T. ) ;
#38114=DIRECTION ( 'NONE',  ( 0.000000000000000000, -0.7071067811865461294, -0.7071067811865487940 ) ) ;
#38167=CARTESIAN_POINT ( 'NONE',  ( 58.00000000000000000, 8.437969416220405915E-15, -2.995852231480068572E-16 ) ) ;
#38259=FACE_BOUND ( 'NONE', #9621, .T. ) ;
#38285=CARTESIAN_POINT ( 'NONE',  ( 4.999999999999983125, 80.00000000000001421, 2.649999999999992806 ) ) ;
#38345=DIRECTION ( 'NONE',  ( -1.000000000000000000, -3.135800716341489291E-16, 1.298891185607901956E-16 ) ) ;
#38456=CARTESIAN_POINT ( 'NONE',  ( 53.14999999999999858, 15.50000000000000711, 1.598617295522242905E-15 ) ) ;
#38485=CARTESIAN_POINT ( 'NONE',  ( 52.49655874117198096, 15.40126909844818748, -1.751009045720654189 ) ) ;
#38488=FACE_BOUND ( 'NONE', #7362, .T. ) ;
#38524=CARTESIAN_POINT ( 'NONE',  ( 50.15454924916686252, 15.27473315039759427, 2.633196453571728490 ) ) ;
#38563=FACE_BOUND ( 'NONE', #13040, .T. ) ;
#38584=EDGE_CURVE ( 'NONE', #58558, #28153, #17742, .T. ) ;
#38595=CARTESIAN_POINT ( 'NONE',  ( 4.999999999999983125, 80.00000000000001421, -3.562970397116383044E-32 ) ) ;
#38608=AXIS2_PLACEMENT_3D ( 'NONE', #32027, #60498, #54877 ) ;
#38625=PRODUCT_DEFINITION_CONTEXT ( 'detailed design', #2759, 'design' ) ;
#38654=ORIENTED_EDGE ( 'NONE', *, *, #16131, .F. ) ;
#38658=LINE ( 'NONE', #57712, #23468 ) ;
#38688=CARTESIAN_POINT ( 'NONE',  ( 5.000000000000012434, -80.00000000000001421, -2.649999999999992806 ) ) ;
#38742=CARTESIAN_POINT ( 'NONE',  ( 4.999999999999996447, 2.650000000000831246, -79.99999999999998579 ) ) ;
#38780=CARTESIAN_POINT ( 'NONE',  ( 50.50000000000000000, 15.27178771460631168, -2.649999999999992806 ) ) ;
#38800=CARTESIAN_POINT ( 'NONE',  ( 52.79985433695213715, 15.44369255379625372, -1.327983408852838387 ) ) ;
#38807=DIRECTION ( 'NONE',  ( 0.000000000000000000, 1.000000000000000000, 0.000000000000000000 ) ) ;
#38858=EDGE_CURVE ( 'NONE', #36643, #28137, #56713, .T. ) ;
#38902=ORIENTED_EDGE ( 'NONE', *, *, #59760, .T. ) ;
#38904=CARTESIAN_POINT ( 'NONE',  ( 7.999999999999996447, 8.394250489469390599E-13, -80.00000000000001421 ) ) ;
#38908=DIRECTION ( 'NONE',  ( -1.000000000000000000, -0.000000000000000000, 1.925929944387235853E-32 ) ) ;
#38924=VECTOR ( 'NONE', #42217, 1000.000000000000000 ) ;
#38963=CARTESIAN_POINT ( 'NONE',  ( 48.74944754206161690, 12.34007061358912871, 1.996972717666336550 ) ) ;
#39002=CARTESIAN_POINT ( 'NONE',  ( 43.00000000000000000, 0.000000000000000000, 0.000000000000000000 ) ) ;
#39020=LINE ( 'NONE', #28974, #53150 ) ;
#39054=ORIENTED_EDGE ( 'NONE', *, *, #49536, .T. ) ;
#39069=EDGE_CURVE ( 'NONE', #57986, #12452, #11764, .T. ) ;
#39113=CARTESIAN_POINT ( 'NONE',  ( 8.000000000000000000, 0.000000000000000000, 0.000000000000000000 ) ) ;
#39269=ORIENTED_EDGE ( 'NONE', *, *, #55010, .T. ) ;
#39300=ADVANCED_FACE ( 'NONE', ( #7318, #26447 ), #17070, .F. ) ;
#39380=EDGE_CURVE ( 'NONE', #29507, #13900, #735, .T. ) ;
#39405=EDGE_CURVE ( 'NONE', #20457, #22596, #13788, .T. ) ;
#39410=ORIENTED_EDGE ( 'NONE', *, *, #47396, .T. ) ;
#39531=CIRCLE ( 'NONE', #24513, 2.649999999999999467 ) ;
#39536=DIRECTION ( 'NONE',  ( 1.836766033387207149E-16, -1.000000000000000000, 0.000000000000000000 ) ) ;
#39576=CARTESIAN_POINT ( 'NONE',  ( 50.15363872391542799, 12.21587082446438188, 2.649999999999994138 ) ) ;
#39841=CARTESIAN_POINT ( 'NONE',  ( 50.84822255766327004, 12.21965688190746491, -2.632713613759657623 ) ) ;
#39866=CIRCLE ( 'NONE', #31840, 2.649999999999997691 ) ;
#39928=DIRECTION ( 'NONE',  ( 0.000000000000000000, 1.000000000000000000, 0.000000000000000000 ) ) ;
#39951=ORIENTED_EDGE ( 'NONE', *, *, #22995, .T. ) ;
#39975=CARTESIAN_POINT ( 'NONE',  ( 43.00000000000000000, 0.000000000000000000, 0.000000000000000000 ) ) ;
#40008=FACE_OUTER_BOUND ( 'NONE', #48225, .T. ) ;
#40086=CARTESIAN_POINT ( 'NONE',  ( 47.85000000000001563, 15.50000000000001243, 0.1751081065780700774 ) ) ;
#40159=CARTESIAN_POINT ( 'NONE',  ( 5.000000000000010658, -72.00000000000002842, 8.817456953860944867E-15 ) ) ;
#40166=LINE ( 'NONE', #6259, #49861 ) ;
#40207=CARTESIAN_POINT ( 'NONE',  ( 49.32549503994585649, 12.27117319987102917, 2.381776070573418558 ) ) ;
#40432=CARTESIAN_POINT ( 'NONE',  ( 7.999999999999986677, 56.56854249492450037, -56.56854249492312192 ) ) ;
#40449=CARTESIAN_POINT ( 'NONE',  ( 51.82890873906638518, 12.28711123495430790, -2.299226249064501015 ) ) ;
#40479=FACE_OUTER_BOUND ( 'NONE', #25999, .T. ) ;
#40642=CARTESIAN_POINT ( 'NONE',  ( 40.00000000000001421, -72.00000000000001421, 8.817456953860944867E-15 ) ) ;
#40674=CARTESIAN_POINT ( 'NONE',  ( 4.999999999999996447, 2.649999999999721023, 80.00000000000002842 ) ) ;
#40678=EDGE_LOOP ( 'NONE', ( #8192, #30295 ) ) ;
#40706=LINE ( 'NONE', #59779, #46249 ) ;
#40847=EDGE_CURVE ( 'NONE', #54373, #14724, #16581, .T. ) ;
#40875=VERTEX_POINT ( 'NONE', #1258 ) ;
#40948=CARTESIAN_POINT ( 'NONE',  ( 40.00000000000000000, 0.000000000000000000, 0.000000000000000000 ) ) ;
#40986=EDGE_CURVE ( 'NONE', #28137, #36643, #20707, .T. ) ;
#41015=SURFACE_STYLE_USAGE ( .BOTH. , #21876 ) ;
#41127=CARTESIAN_POINT ( 'NONE',  ( 47.98570199392409563, 12.47176666825323288, -0.8548734444802772448 ) ) ;
#41174=UNCERTAINTY_MEASURE_WITH_UNIT (LENGTH_MEASURE( 1.000000000000000082E-05 ), #17423, 'distance_accuracy_value', 'NONE');
#41254=FACE_OUTER_BOUND ( 'NONE', #7103, .T. ) ;
#41340=DIRECTION ( 'NONE',  ( -1.000000000000000000, -1.836909530733580185E-16, 1.836909530733574022E-16 ) ) ;
#41402=DIRECTION ( 'NONE',  ( 0.000000000000000000, 0.7071067811865540120, -0.7071067811865409114 ) ) ;
#41410=EDGE_LOOP ( 'NONE', ( #58425, #53444, #59947, #39951 ) ) ;
#41538=AXIS2_PLACEMENT_3D ( 'NONE', #40948, #17117, #7686 ) ;
#41559=CYLINDRICAL_SURFACE ( 'NONE', #47933, 2.649999999999992806 ) ;
#41688=DIRECTION ( 'NONE',  ( 0.000000000000000000, -1.000000000000000000, 0.000000000000000000 ) ) ;
#41696=CARTESIAN_POINT ( 'NONE',  ( 4.999999999999996447, 2.650000000000838352, -79.99999999999998579 ) ) ;
#41750=CARTESIAN_POINT ( 'NONE',  ( 43.00000000000000000, 2.549224068967256441E-30, 75.00000000000001421 ) ) ;
#41751=DIRECTION ( 'NONE',  ( -1.850371707708593823E-16, 1.000000000000000000, 0.000000000000000000 ) ) ;
#41805=AXIS2_PLACEMENT_3D ( 'NONE', #52895, #42297, #56663 ) ;
#41917=AXIS2_PLACEMENT_3D ( 'NONE', #3750, #42020, #41402 ) ;
#41980=EDGE_LOOP ( 'NONE', ( #9367, #26048 ) ) ;
#42020=DIRECTION ( 'NONE',  ( -1.000000000000000000, -3.135800716341471541E-16, -1.298891185607920445E-16 ) ) ;
#42053=DIRECTION ( 'NONE',  ( -3.273063162220399693E-16, 1.000000000000000000, 1.047380211910527902E-14 ) ) ;
#42096=DIRECTION ( 'NONE',  ( 1.836766033387207149E-16, -1.000000000000000000, 0.000000000000000000 ) ) ;
#42116=ORIENTED_EDGE ( 'NONE', *, *, #55151, .F. ) ;
#42125=DIRECTION ( 'NONE',  ( -1.836909530733573776E-16, 1.000000000000000000, 0.000000000000000000 ) ) ;
#42217=DIRECTION ( 'NONE',  ( -0.000000000000000000, -1.000000000000000000, -0.000000000000000000 ) ) ;
#42222=CARTESIAN_POINT ( 'NONE',  ( 5.000000000000012434, -80.00000000000001421, -1.569632904675596344E-31 ) ) ;
#42246=CARTESIAN_POINT ( 'NONE',  ( 47.85000000000000853, 15.50000000000000711, -0.1749776157412613053 ) ) ;
#42289=ORIENTED_EDGE ( 'NONE', *, *, #59918, .T. ) ;
#42297=DIRECTION ( 'NONE',  ( -1.000000000000000000, -5.380183451256491399E-17, -1.298891185607892835E-16 ) ) ;
#42334=AXIS2_PLACEMENT_3D ( 'NONE', #51148, #8233, #60854 ) ;
#42351=CARTESIAN_POINT ( 'NONE',  ( 8.000000000000007105, -58.44237546506844438, 54.69470952477916370 ) ) ;
#42434=DIRECTION ( 'NONE',  ( -1.000000000000000000, -0.000000000000000000, 1.925929944387235853E-32 ) ) ;
#42555=CYLINDRICAL_SURFACE ( 'NONE', #2160, 2.649999999999992806 ) ;
#42638=FACE_BOUND ( 'NONE', #41980, .T. ) ;
#42738=LINE ( 'NONE', #23924, #27437 ) ;
#42820=LINE ( 'NONE', #38742, #7492 ) ;
#42860=CARTESIAN_POINT ( 'NONE',  ( 48.11856151137951088, 15.45621073281055402, -1.175286366004017813 ) ) ;
#42904=ORIENTED_EDGE ( 'NONE', *, *, #38858, .F. ) ;
#43016=DIRECTION ( 'NONE',  ( 1.000000000000000000, 1.836909530733573776E-16, -1.925929944387235853E-32 ) ) ;
#43044=VERTEX_POINT ( 'NONE', #40674 ) ;
#43108=EDGE_CURVE ( 'NONE', #60397, #14724, #52809, .T. ) ;
#43156=CARTESIAN_POINT ( 'NONE',  ( 53.13262160778436538, 15.49700215203310272, 0.3490842977376169554 ) ) ;
#43166=CYLINDRICAL_SURFACE ( 'NONE', #5468, 85.00000000000001421 ) ;
#43181=EDGE_CURVE ( 'NONE', #8457, #29507, #34043, .T. ) ;
#43341=MECHANICAL_DESIGN_GEOMETRIC_PRESENTATION_REPRESENTATION('',(#25292),#46333);
#43383=ADVANCED_FACE ( 'NONE', ( #51189 ), #2024, .F. ) ;
#43411=EDGE_LOOP ( 'NONE', ( #50477, #3688, #5912, #22679 ) ) ;
#43477=CARTESIAN_POINT ( 'NONE',  ( 49.16403548792207090, 15.32681626569766209, -2.314452977059477945 ) ) ;
#43500=FACE_BOUND ( 'NONE', #59327, .T. ) ;
#43513=EDGE_LOOP ( 'NONE', ( #59032, #14136 ) ) ;
#43524=CARTESIAN_POINT ( 'NONE',  ( 5.000000000000007994, -54.69470952477895054, -58.44237546506863623 ) ) ;
#43529=AXIS2_PLACEMENT_3D ( 'NONE', #7418, #60658, #16538 ) ;
#43571=FACE_BOUND ( 'NONE', #44636, .T. ) ;
#43614=VECTOR ( 'NONE', #11059, 1000.000000000000000 ) ;
#43698=CARTESIAN_POINT ( 'NONE',  ( 47.85000000000000853, 15.50000000000000711, 1.598617397282144235E-15 ) ) ;
#43742=EDGE_LOOP ( 'NONE', ( #7504, #51926 ) ) ;
#43754=DIRECTION ( 'NONE',  ( -1.000000000000000000, -1.836909530733554547E-16, -1.836909530733573529E-16 ) ) ;
#43772=CYLINDRICAL_SURFACE ( 'NONE', #1778, 2.649999999999992806 ) ;
#43806=CARTESIAN_POINT ( 'NONE',  ( 7.999999999999986677, 58.44237546506807490, 54.69470952477956871 ) ) ;
#43817=CARTESIAN_POINT ( 'NONE',  ( 51.82869273375258956, 15.32880936072750799, -2.299358913708370533 ) ) ;
#43889=AXIS2_PLACEMENT_3D ( 'NONE', #8716, #56015, #60392 ) ;
#43893=FACE_BOUND ( 'NONE', #21209, .T. ) ;
#43922=EDGE_LOOP ( 'NONE', ( #60782, #6604, #21810, #53740 ) ) ;
#43928=DIRECTION ( 'NONE',  ( 0.000000000000000000, 0.000000000000000000, 1.000000000000000000 ) ) ;
#44022=ADVANCED_FACE ( 'NONE', ( #25394 ), #57966, .F. ) ;
#44026=EDGE_CURVE ( 'NONE', #28153, #44393, #12247, .T. ) ;
#44082=VECTOR ( 'NONE', #37479, 1000.000000000000000 ) ;
#44106=EDGE_LOOP ( 'NONE', ( #11591, #31603, #59558, #56879 ) ) ;
#44230=CARTESIAN_POINT ( 'NONE',  ( 51.35512545846777499, 12.24472452707400549, 2.514220983385977881 ) ) ;
#44250=AXIS2_PLACEMENT_3D ( 'NONE', #27822, #3988, #3375 ) ;
#44279=CARTESIAN_POINT ( 'NONE',  ( 47.93443732600252360, 12.48232846285511677, -0.6858480285855463876 ) ) ;
#44358=DIRECTION ( 'NONE',  ( -1.000000000000000000, -0.000000000000000000, -0.000000000000000000 ) ) ;
#44393=VERTEX_POINT ( 'NONE', #40642 ) ;
#44494=CARTESIAN_POINT ( 'NONE',  ( 43.00000000000000000, 0.000000000000000000, 75.00000000000001421 ) ) ;
#44498=CIRCLE ( 'NONE', #449, 12.50000000000000000 ) ;
#44525=ADVANCED_FACE ( 'NONE', ( #41254 ), #41559, .F. ) ;
#44537=CARTESIAN_POINT ( 'NONE',  ( 51.67535452159865628, 12.27124677633248240, 2.381404722338403168 ) ) ;
#44565=DIRECTION ( 'NONE',  ( 1.000000000000000000, 1.836909530733573776E-16, -1.925929944387235853E-32 ) ) ;
#44618=DIRECTION ( 'NONE',  ( -1.000000000000000000, -0.000000000000000000, -0.000000000000000000 ) ) ;
#44636=EDGE_LOOP ( 'NONE', ( #49723, #9996 ) ) ;
#44644=AXIS2_PLACEMENT_3D ( 'NONE', #34667, #59062, #11474 ) ;
#44662=CYLINDRICAL_SURFACE ( 'NONE', #50734, 2.649999999999992806 ) ;
#44734=FACE_OUTER_BOUND ( 'NONE', #49388, .T. ) ;
#45066=ORIENTED_EDGE ( 'NONE', *, *, #33396, .F. ) ;
#45109=ORIENTED_EDGE ( 'NONE', *, *, #6685, .F. ) ;
#45126=EDGE_LOOP ( 'NONE', ( #36009, #51459 ) ) ;
#45138=ORIENTED_EDGE ( 'NONE', *, *, #25236, .T. ) ;
#45187=EDGE_CURVE ( 'NONE', #23359, #43044, #28967, .T. ) ;
#45208=CARTESIAN_POINT ( 'NONE',  ( 49.64102424810503322, 12.24500408462137813, -2.512856703132412495 ) ) ;
#45273=DIRECTION ( 'NONE',  ( 0.000000000000000000, 0.000000000000000000, 1.000000000000000000 ) ) ;
#45371=ORIENTED_EDGE ( 'NONE', *, *, #5146, .F. ) ;
#45409=EDGE_CURVE ( 'NONE', #4875, #50598, #11504, .T. ) ;
#45538=AXIS2_PLACEMENT_3D ( 'NONE', #54387, #1773, #35641 ) ;
#45608=CYLINDRICAL_SURFACE ( 'NONE', #45851, 2.649999999999992806 ) ;
#45683=AXIS2_PLACEMENT_3D ( 'NONE', #39002, #44618, #24880 ) ;
#45705=CARTESIAN_POINT ( 'NONE',  ( 58.00000000000000000, 15.50000000000001066, 1.598617315530391440E-15 ) ) ;
#45799=ADVANCED_FACE ( 'NONE', ( #32085, #27683 ), #51162, .T. ) ;
#45851=AXIS2_PLACEMENT_3D ( 'NONE', #36213, #55278, #9529 ) ;
#45953=ORIENTED_EDGE ( 'NONE', *, *, #52615, .F. ) ;
#46022=CARTESIAN_POINT ( 'NONE',  ( 4.999999999999986677, 56.56854249492371878, 56.56854249492391062 ) ) ;
#46032=CARTESIAN_POINT ( 'NONE',  ( 5.000000000000012434, -80.00000000000001421, -2.649999999999999467 ) ) ;
#46180=ORIENTED_EDGE ( 'NONE', *, *, #40847, .T. ) ;
#46233=DIRECTION ( 'NONE',  ( -1.000000000000000000, -5.380183451256670742E-17, 1.298891185607911324E-16 ) ) ;
#46245=ORIENTED_EDGE ( 'NONE', *, *, #43181, .F. ) ;
#46249=VECTOR ( 'NONE', #59146, 1000.000000000000000 ) ;
#46316=DIRECTION ( 'NONE',  ( -1.000000000000000000, -5.380183451256670742E-17, 1.298891185607911324E-16 ) ) ;
#46333=( GEOMETRIC_REPRESENTATION_CONTEXT ( 3 ) GLOBAL_UNCERTAINTY_ASSIGNED_CONTEXT ( ( #41174 ) ) GLOBAL_UNIT_ASSIGNED_CONTEXT ( ( #17423, #10185, #53383 ) ) REPRESENTATION_CONTEXT ( 'NONE', 'WORKASPACE' ) );
#46380=DIRECTION ( 'NONE',  ( -1.000000000000000000, -0.000000000000000000, -0.000000000000000000 ) ) ;
#46444=CARTESIAN_POINT ( 'NONE',  ( 43.00000000000000000, 0.000000000000000000, 0.000000000000000000 ) ) ;
#46478=CYLINDRICAL_SURFACE ( 'NONE', #42334, 2.649999999999997691 ) ;
#46488=ADVANCED_FACE ( 'NONE', ( #25526 ), #44662, .F. ) ;
#46493=CARTESIAN_POINT ( 'NONE',  ( 58.00000000000000000, 8.437969416220405915E-15, -2.995852231480068572E-16 ) ) ;
#46519=CIRCLE ( 'NONE', #27498, 2.649999999999997691 ) ;
#46522=CARTESIAN_POINT ( 'NONE',  ( 7.999999999999996447, 1.469527624586858429E-15, -1.540743955509788245E-31 ) ) ;
#46586=ORIENTED_EDGE ( 'NONE', *, *, #22838, .T. ) ;
#46598=FACE_OUTER_BOUND ( 'NONE', #60864, .T. ) ;
#46628=LINE ( 'NONE', #61003, #17782 ) ;
#46688=CARTESIAN_POINT ( 'NONE',  ( 58.00000000000000000, 8.437969416220405915E-15, -2.995852231480068572E-16 ) ) ;
#46692=CIRCLE ( 'NONE', #1658, 2.649999999999997691 ) ;
#46735=AXIS2_PLACEMENT_3D ( 'NONE', #58170, #19683, #38807 ) ;
#46861=DIRECTION ( 'NONE',  ( 0.000000000000000000, 1.000000000000000000, 0.000000000000000000 ) ) ;
#46878=SURFACE_STYLE_FILL_AREA ( #4525 ) ;
#46921=EDGE_LOOP ( 'NONE', ( #36241, #26052, #39054, #5918 ) ) ;
#46927=AXIS2_PLACEMENT_3D ( 'NONE', #26157, #2960, #21154 ) ;
#47153=CARTESIAN_POINT ( 'NONE',  ( 5.000000000000007994, -56.56854249492331377, -56.56854249492430142 ) ) ;
#47253=CARTESIAN_POINT ( 'NONE',  ( 51.67657445772706382, 15.31620728304649326, -2.380828478538471238 ) ) ;
#47288=CARTESIAN_POINT ( 'NONE',  ( 48.50459710310596506, 15.40111741581167593, 1.752346893213588386 ) ) ;
#47320=CIRCLE ( 'NONE', #26297, 2.649999999999997691 ) ;
#47396=EDGE_CURVE ( 'NONE', #15197, #96, #56808, .T. ) ;
#47488=DIRECTION ( 'NONE',  ( -1.000000000000000000, -1.836909530733573776E-16, 1.103352205049209901E-32 ) ) ;
#47498=ORIENTED_EDGE ( 'NONE', *, *, #28082, .T. ) ;
#47560=DIRECTION ( 'NONE',  ( 0.000000000000000000, 1.000000000000000000, 0.000000000000000000 ) ) ;
#47607=EDGE_CURVE ( 'NONE', #49238, #50555, #1757, .T. ) ;
#47762=DIRECTION ( 'NONE',  ( -1.000000000000000000, -3.135800716341471541E-16, -1.298891185607920445E-16 ) ) ;
#47849=CARTESIAN_POINT ( 'NONE',  ( 50.67307810846496352, 15.27178771460631346, 2.649999999999992806 ) ) ;
#47856=CIRCLE ( 'NONE', #4788, 2.649999999999999467 ) ;
#47858=CARTESIAN_POINT ( 'NONE',  ( 48.39222823129596662, 15.41626216437607155, -1.615489271240708291 ) ) ;
#47876=CARTESIAN_POINT ( 'NONE',  ( 51.18719699018952696, 15.28630115564075354, -2.565184398965006718 ) ) ;
#47896=DIRECTION ( 'NONE',  ( 0.000000000000000000, 0.000000000000000000, 1.000000000000000000 ) ) ;
#47933=AXIS2_PLACEMENT_3D ( 'NONE', #18365, #17737, #23059 ) ;
#47939=CARTESIAN_POINT ( 'NONE',  ( 8.000000000000000000, 9.184850993605147156E-15, -75.00000000000001421 ) ) ;
#47947=AXIS2_PLACEMENT_3D ( 'NONE', #32379, #27980, #4147 ) ;
#48012=UNCERTAINTY_MEASURE_WITH_UNIT (LENGTH_MEASURE( 1.000000000000000082E-05 ), #11240, 'distance_accuracy_value', 'NONE');
#48013=EDGE_LOOP ( 'NONE', ( #57383, #48193, #3517, #24894 ) ) ;
#48038=CARTESIAN_POINT ( 'NONE',  ( 5.000000000000007994, -56.56854249492410958, 56.56854249492351983 ) ) ;
#48159=CARTESIAN_POINT ( 'NONE',  ( 4.999999999999986677, 54.69470952478017978, -58.44237546506749226 ) ) ;
#48193=ORIENTED_EDGE ( 'NONE', *, *, #57466, .T. ) ;
#48225=EDGE_LOOP ( 'NONE', ( #33633, #31333, #42904, #42116 ) ) ;
#48285=DIRECTION ( 'NONE',  ( -1.000000000000000000, -0.000000000000000000, 1.925929944387235853E-32 ) ) ;
#48335=CARTESIAN_POINT ( 'NONE',  ( 48.11999735391012223, 12.44538514811858221, 1.178318479186655887 ) ) ;
#48403=ORIENTED_EDGE ( 'NONE', *, *, #60454, .F. ) ;
#48408=DIRECTION ( 'NONE',  ( -1.000000000000000000, -1.836909530733573529E-16, 1.361838123766461297E-32 ) ) ;
#48476=DIRECTION ( 'NONE',  ( -1.000000000000000000, -1.836909530733573776E-16, 1.925929944387235853E-32 ) ) ;
#48502=DIRECTION ( 'NONE',  ( -3.273063162220391312E-16, 1.000000000000000000, 1.047380211910525220E-14 ) ) ;
#48508=EDGE_CURVE ( 'NONE', #60397, #49193, #10385, .T. ) ;
#48587=EDGE_CURVE ( 'NONE', #50941, #37408, #47856, .T. ) ;
#48771=AXIS2_PLACEMENT_3D ( 'NONE', #5399, #28919, #9196 ) ;
#48858=VERTEX_POINT ( 'NONE', #24330 ) ;
#48859=AXIS2_PLACEMENT_3D ( 'NONE', #57780, #47488, #18677 ) ;
#48894=CARTESIAN_POINT ( 'NONE',  ( 52.60679555148794861, 12.39585383992677059, 1.616669970113162824 ) ) ;
#48967=ORIENTED_EDGE ( 'NONE', *, *, #48587, .F. ) ;
#49011=ADVANCED_FACE ( 'NONE', ( #50586 ), #45608, .F. ) ;
#49051=DIRECTION ( 'NONE',  ( -1.000000000000000000, -1.836909530733573776E-16, 1.925929944387235853E-32 ) ) ;
#49130=ORIENTED_EDGE ( 'NONE', *, *, #9848, .F. ) ;
#49131=DIRECTION ( 'NONE',  ( 0.000000000000000000, -0.7071067811865435759, -0.7071067811865514585 ) ) ;
#49182=ORIENTED_EDGE ( 'NONE', *, *, #8269, .T. ) ;
#49183=DIRECTION ( 'NONE',  ( 0.000000000000000000, -0.7071067811865553443, 0.7071067811865395791 ) ) ;
#49193=VERTEX_POINT ( 'NONE', #43698 ) ;
#49238=VERTEX_POINT ( 'NONE', #41696 ) ;
#49265=ORIENTED_EDGE ( 'NONE', *, *, #6210, .T. ) ;
#49367=CYLINDRICAL_SURFACE ( 'NONE', #44644, 12.50000000000000000 ) ;
#49388=EDGE_LOOP ( 'NONE', ( #51540, #15073 ) ) ;
#49413=ORIENTED_EDGE ( 'NONE', *, *, #30276, .T. ) ;
#49506=CARTESIAN_POINT ( 'NONE',  ( 50.67322615039200429, 12.21587082446438011, 2.649999999999992362 ) ) ;
#49536=EDGE_CURVE ( 'NONE', #26981, #24288, #39866, .T. ) ;
#49614=EDGE_CURVE ( 'NONE', #26701, #9789, #27492, .T. ) ;
#49682=CARTESIAN_POINT ( 'NONE',  ( 8.000000000000000000, -2.549224068967256091E-30, 75.00000000000001421 ) ) ;
#49703=CARTESIAN_POINT ( 'NONE',  ( 8.000000000000012434, -85.00000000000001421, -1.540743955509788245E-31 ) ) ;
#49723=ORIENTED_EDGE ( 'NONE', *, *, #6356, .F. ) ;
#49819=CARTESIAN_POINT ( 'NONE',  ( 52.25241694927984071, 12.34033889370408232, -1.995302726669112570 ) ) ;
#49861=VECTOR ( 'NONE', #16318, 1000.000000000000000 ) ;
#49872=STYLED_ITEM ( 'NONE', ( #36921 ), #34065 ) ;
#49949=CARTESIAN_POINT ( 'NONE',  ( 43.00000000000000000, 0.000000000000000000, 0.000000000000000000 ) ) ;
#49972=VECTOR ( 'NONE', #35708, 1000.000000000000000 ) ;
#50025=ORIENTED_EDGE ( 'NONE', *, *, #31544, .F. ) ;
#50055=CARTESIAN_POINT ( 'NONE',  ( 4.999999999999998224, -2.650000000000277911, 80.00000000000000000 ) ) ;
#50076=DIRECTION ( 'NONE',  ( 0.000000000000000000, -0.7071067811865487940, 0.7071067811865461294 ) ) ;
#50186=CARTESIAN_POINT ( 'NONE',  ( 48.86838059950356694, 12.32200637394865161, -2.116332808070153337 ) ) ;
#50194=FACE_OUTER_BOUND ( 'NONE', #31641, .T. ) ;
#50217=DIRECTION ( 'NONE',  ( 0.000000000000000000, -0.7071067811865487940, 0.7071067811865461294 ) ) ;
#50221=DIRECTION ( 'NONE',  ( -1.000000000000000000, -5.380183451256491399E-17, -1.298891185607892835E-16 ) ) ;
#50273=PRODUCT_DEFINITION_SHAPE ( 'NONE', 'NONE',  #3771 ) ;
#50293=VECTOR ( 'NONE', #38908, 1000.000000000000000 ) ;
#50303=EDGE_LOOP ( 'NONE', ( #51374, #59504, #5405, #11292 ) ) ;
#50477=ORIENTED_EDGE ( 'NONE', *, *, #19260, .F. ) ;
#50487=CARTESIAN_POINT ( 'NONE',  ( 48.19965373053142343, 12.43020942110654659, -1.327029891807659512 ) ) ;
#50547=AXIS2_PLACEMENT_3D ( 'NONE', #31143, #60559, #12681 ) ;
#50555=VERTEX_POINT ( 'NONE', #10979 ) ;
#50567=VERTEX_POINT ( 'NONE', #58551 ) ;
#50586=FACE_OUTER_BOUND ( 'NONE', #11819, .T. ) ;
#50598=VERTEX_POINT ( 'NONE', #7471 ) ;
#50734=AXIS2_PLACEMENT_3D ( 'NONE', #54317, #36188, #25840 ) ;
#50819=AXIS2_PLACEMENT_3D ( 'NONE', #49949, #26136, #45273 ) ;
#50823=DIRECTION ( 'NONE',  ( -1.000000000000000000, -3.673819061467147552E-16, 1.925929944387235306E-32 ) ) ;
#50941=VERTEX_POINT ( 'NONE', #25600 ) ;
#51075=ORIENTED_EDGE ( 'NONE', *, *, #18019, .F. ) ;
#51148=CARTESIAN_POINT ( 'NONE',  ( 4.999999999999986677, 56.56854249492371878, 56.56854249492391062 ) ) ;
#51162=PLANE ( 'NONE',  #14987 ) ;
#51189=FACE_OUTER_BOUND ( 'NONE', #44106, .T. ) ;
#51220=FACE_BOUND ( 'NONE', #17874, .T. ) ;
#51310=DIRECTION ( 'NONE',  ( 3.273063162220391312E-16, -1.000000000000000000, -5.236901059552626099E-15 ) ) ;
#51354=LINE ( 'NONE', #32274, #14824 ) ;
#51359=DIRECTION ( 'NONE',  ( -1.000000000000000000, -1.836909530733573776E-16, 1.925929944387235306E-32 ) ) ;
#51374=ORIENTED_EDGE ( 'NONE', *, *, #61843, .F. ) ;
#51378=CARTESIAN_POINT ( 'NONE',  ( 8.000000000000007105, -54.69470952477976766, 58.44237546506786884 ) ) ;
#51390=ORIENTED_EDGE ( 'NONE', *, *, #47396, .F. ) ;
#51413=DIRECTION ( 'NONE',  ( 0.000000000000000000, 0.000000000000000000, 1.000000000000000000 ) ) ;
#51459=ORIENTED_EDGE ( 'NONE', *, *, #17947, .T. ) ;
#51513=AXIS2_PLACEMENT_3D ( 'NONE', #38167, #37862, #33457 ) ;
#51540=ORIENTED_EDGE ( 'NONE', *, *, #33800, .F. ) ;
#51564=CARTESIAN_POINT ( 'NONE',  ( 40.00000000000000000, 4.422198837962619519E-47, 12.50000000000000000 ) ) ;
#51578=CIRCLE ( 'NONE', #17575, 2.649999999999999467 ) ;
#51597=EDGE_CURVE ( 'NONE', #32701, #50567, #36421, .T. ) ;
#51752=AXIS2_PLACEMENT_3D ( 'NONE', #48038, #38345, #19848 ) ;
#51926=ORIENTED_EDGE ( 'NONE', *, *, #49536, .F. ) ;
#52059=FACE_OUTER_BOUND ( 'NONE', #34053, .T. ) ;
#52169=ORIENTED_EDGE ( 'NONE', *, *, #48587, .T. ) ;
#52306=AXIS2_PLACEMENT_3D ( 'NONE', #59860, #25733, #16979 ) ;
#52340=LINE ( 'NONE', #52960, #60513 ) ;
#52414=DIRECTION ( 'NONE',  ( -1.000000000000000000, -0.000000000000000000, -0.000000000000000000 ) ) ;
#52468=LINE ( 'NONE', #14597, #44082 ) ;
#52519=CARTESIAN_POINT ( 'NONE',  ( 51.18913332871307631, 15.28638276972803034, 2.564700684161830502 ) ) ;
#52568=AXIS2_PLACEMENT_3D ( 'NONE', #17059, #55545, #60244 ) ;
#52580=DIRECTION ( 'NONE',  ( -1.000000000000000000, -3.135800716341471541E-16, -1.298891185607920445E-16 ) ) ;
#52615=EDGE_CURVE ( 'NONE', #37408, #50941, #20436, .T. ) ;
#52774=ORIENTED_EDGE ( 'NONE', *, *, #49614, .T. ) ;
#52809=LINE ( 'NONE', #29014, #38924 ) ;
#52835=CARTESIAN_POINT ( 'NONE',  ( 52.79844894553458801, 15.44348932695818810, 1.330174488105935193 ) ) ;
#52847=CARTESIAN_POINT ( 'NONE',  ( 49.64180998113290144, 15.29505603208808395, -2.513117253861154143 ) ) ;
#52853=DIRECTION ( 'NONE',  ( -1.000000000000000000, -1.836909530733573776E-16, 1.925929944387235853E-32 ) ) ;
#52895=CARTESIAN_POINT ( 'NONE',  ( 4.999999999999986677, 56.56854249492450037, -56.56854249492312192 ) ) ;
#52960=CARTESIAN_POINT ( 'NONE',  ( 58.00000000000000000, 15.50000000000000888, 1.598617315530390651E-15 ) ) ;
#53022=CARTESIAN_POINT ( 'NONE',  ( 49.17070544691794964, 12.28715003449873855, 2.299028855467196486 ) ) ;
#53150=VECTOR ( 'NONE', #61538, 1000.000000000000000 ) ;
#53176=ORIENTED_EDGE ( 'NONE', *, *, #40986, .T. ) ;
#53240=ORIENTED_EDGE ( 'NONE', *, *, #6561, .T. ) ;
#53383=( NAMED_UNIT ( * ) SI_UNIT ( $, .STERADIAN. ) SOLID_ANGLE_UNIT ( ) );
#53444=ORIENTED_EDGE ( 'NONE', *, *, #51597, .F. ) ;
#53558=EDGE_LOOP ( 'NONE', ( #51390, #8259, #231, #51075 ) ) ;
#53580=ADVANCED_FACE ( 'NONE', ( #55703 ), #32236, .F. ) ;
#53740=ORIENTED_EDGE ( 'NONE', *, *, #30404, .F. ) ;
#53773=ADVANCED_FACE ( 'NONE', ( #28138, #33476, #19370, #38488, #33790, #9971, #43500, #15904, #30915, #44734 ), #11203, .F. ) ;
#53882=CARTESIAN_POINT ( 'NONE',  ( 52.79846469724564884, 12.42986503907192564, 1.330138836193681895 ) ) ;
#53888=CYLINDRICAL_SURFACE ( 'NONE', #2822, 15.50000000000000000 ) ;
#53933=LINE ( 'NONE', #1013, #43614 ) ;
#54078=CARTESIAN_POINT ( 'NONE',  ( 5.000000000000007994, -56.56854249492331377, -56.56854249492430142 ) ) ;
#54113=CARTESIAN_POINT ( 'NONE',  ( 7.999999999999986677, 58.44237546506882808, -54.69470952477875869 ) ) ;
#54184=CARTESIAN_POINT ( 'NONE',  ( 53.13270191851064084, 12.49630009966210054, 0.3485413523074348818 ) ) ;
#54266=CARTESIAN_POINT ( 'NONE',  ( 5.000000000000012434, -80.00000000000001421, 2.649999999999992806 ) ) ;
#54317=CARTESIAN_POINT ( 'NONE',  ( 4.999999999999997335, -2.784000523420839360E-13, 80.00000000000001421 ) ) ;
#54330=AXIS2_PLACEMENT_3D ( 'NONE', #46522, #17389, #55577 ) ;
#54361=EDGE_CURVE ( 'NONE', #14724, #54373, #21968, .T. ) ;
#54373=VERTEX_POINT ( 'NONE', #12002 ) ;
#54384=DIRECTION ( 'NONE',  ( 0.000000000000000000, 0.7071067811865540120, -0.7071067811865409114 ) ) ;
#54387=CARTESIAN_POINT ( 'NONE',  ( 7.999999999999996447, 1.469527624586858429E-15, -1.540743955509788245E-31 ) ) ;
#54491=CARTESIAN_POINT ( 'NONE',  ( 50.84915202508826582, 12.21967388707288471, 2.632638007633139487 ) ) ;
#54525=CARTESIAN_POINT ( 'NONE',  ( 58.00000000000000000, 1.530808498934191127E-15, -12.50000000000000000 ) ) ;
#54673=ORIENTED_EDGE ( 'NONE', *, *, #33324, .T. ) ;
#54819=EDGE_CURVE ( 'NONE', #20457, #49238, #42820, .T. ) ;
#54865=CARTESIAN_POINT ( 'NONE',  ( 48.50340449756345151, 12.37737586902969333, -1.750926327775586211 ) ) ;
#54877=DIRECTION ( 'NONE',  ( 0.000000000000000000, -0.7071067811865449082, -0.7071067811865500152 ) ) ;
#54883=ORIENTED_EDGE ( 'NONE', *, *, #25236, .F. ) ;
#54892=DIRECTION ( 'NONE',  ( 1.000000000000000000, 1.836909530733573776E-16, -1.925929944387235853E-32 ) ) ;
#54912=CARTESIAN_POINT ( 'NONE',  ( 7.999999999999996447, 2.649999999999714806, 80.00000000000002842 ) ) ;
#54937=VECTOR ( 'NONE', #52580, 1000.000000000000000 ) ;
#55010=EDGE_CURVE ( 'NONE', #6447, #16220, #46519, .T. ) ;
#55013=EDGE_LOOP ( 'NONE', ( #3442, #15863 ) ) ;
#55151=EDGE_CURVE ( 'NONE', #59796, #36643, #14236, .T. ) ;
#55278=DIRECTION ( 'NONE',  ( -0.000000000000000000, -1.000000000000000000, -0.000000000000000000 ) ) ;
#55309=ADVANCED_FACE ( 'NONE', ( #50194 ), #12933, .F. ) ;
#55350=VERTEX_POINT ( 'NONE', #41750 ) ;
#55363=( NAMED_UNIT ( * ) SI_UNIT ( $, .STERADIAN. ) SOLID_ANGLE_UNIT ( ) );
#55421=ORIENTED_EDGE ( 'NONE', *, *, #11831, .F. ) ;
#55436=AXIS2_PLACEMENT_3D ( 'NONE', #22317, #32337, #51413 ) ;
#55471=AXIS2_PLACEMENT_3D ( 'NONE', #12036, #31111, #50217 ) ;
#55545=DIRECTION ( 'NONE',  ( -1.000000000000000000, -1.836909530733573776E-16, 1.925929944387235853E-32 ) ) ;
#55577=DIRECTION ( 'NONE',  ( 1.836766033387207149E-16, -1.000000000000000000, 0.000000000000000000 ) ) ;
#55599=CIRCLE ( 'NONE', #52568, 85.00000000000001421 ) ;
#55684=CIRCLE ( 'NONE', #28697, 2.649999999999999467 ) ;
#55703=FACE_OUTER_BOUND ( 'NONE', #48013, .T. ) ;
#55769=DIRECTION ( 'NONE',  ( 1.000000000000000000, 1.836909530733573776E-16, -1.925929944387235853E-32 ) ) ;
#55885=DIRECTION ( 'NONE',  ( -1.000000000000000000, -1.836909530733573776E-16, 1.361838123766442686E-32 ) ) ;
#55890=ORIENTED_EDGE ( 'NONE', *, *, #25179, .T. ) ;
#55916=EDGE_LOOP ( 'NONE', ( #620, #18956 ) ) ;
#56015=DIRECTION ( 'NONE',  ( -1.000000000000000000, -1.836909530733554547E-16, -1.836909530733573529E-16 ) ) ;
#56016=AXIS2_PLACEMENT_3D ( 'NONE', #12880, #7842, #2520 ) ;
#56092=ORIENTED_EDGE ( 'NONE', *, *, #5129, .F. ) ;
#56112=ORIENTED_EDGE ( 'NONE', *, *, #36302, .T. ) ;
#56135=CYLINDRICAL_SURFACE ( 'NONE', #19409, 2.649999999999992806 ) ;
#56281=ADVANCED_FACE ( 'NONE', ( #43893, #37960, #10349, #43571, #38563, #42638, #14139, #38259, #9720, #5 ), #58235, .T. ) ;
#56413=EDGE_LOOP ( 'NONE', ( #9135, #7552, #12653, #2018, #16271 ) ) ;
#56498=CARTESIAN_POINT ( 'NONE',  ( 4.999999999999986677, 58.44237546506807490, 54.69470952477956871 ) ) ;
#56510=EDGE_CURVE ( 'NONE', #12923, #60397, #57528, .T. ) ;
#56573=ADVANCED_FACE ( 'NONE', ( #40008 ), #49367, .F. ) ;
#56603=CARTESIAN_POINT ( 'NONE',  ( 52.49678397332792201, 15.40128748659475377, 1.750934580577085287 ) ) ;
#56663=DIRECTION ( 'NONE',  ( 0.000000000000000000, 0.7071067811865395791, 0.7071067811865553443 ) ) ;
#56672=ORIENTED_EDGE ( 'NONE', *, *, #39380, .T. ) ;
#56713=CIRCLE ( 'NONE', #46735, 12.50000000000000000 ) ;
#56729=DIRECTION ( 'NONE',  ( -1.000000000000000000, -1.836909530733573776E-16, 1.925929944387235853E-32 ) ) ;
#56782=AXIS2_PLACEMENT_3D ( 'NONE', #10532, #49051, #30544 ) ;
#56808=CIRCLE ( 'NONE', #6752, 2.649999999999985700 ) ;
#56879=ORIENTED_EDGE ( 'NONE', *, *, #8861, .F. ) ;
#56910=EDGE_CURVE ( 'NONE', #30745, #4178, #24251, .T. ) ;
#56921=CARTESIAN_POINT ( 'NONE',  ( 49.80938579167644775, 15.28643915577036339, -2.564367652788756669 ) ) ;
#56991=ADVANCED_FACE ( 'NONE', ( #26102 ), #59605, .F. ) ;
#57007=ORIENTED_EDGE ( 'NONE', *, *, #8024, .F. ) ;
#57051=ADVANCED_FACE ( 'NONE', ( #52059 ), #8848, .T. ) ;
#57316=EDGE_LOOP ( 'NONE', ( #54883, #33939 ) ) ;
#57359=ADVANCED_FACE ( 'NONE', ( #60684 ), #43166, .T. ) ;
#57361=CARTESIAN_POINT ( 'NONE',  ( 8.000000000000012434, -80.00000000000001421, -2.649999999999992806 ) ) ;
#57363=ORIENTED_EDGE ( 'NONE', *, *, #59918, .F. ) ;
#57383=ORIENTED_EDGE ( 'NONE', *, *, #60677, .F. ) ;
#57466=EDGE_CURVE ( 'NONE', #50567, #31453, #29047, .T. ) ;
#57506=CARTESIAN_POINT ( 'NONE',  ( 52.11658891626548495, 15.35644817774449145, 2.106865129802042436 ) ) ;
#57527=CARTESIAN_POINT ( 'NONE',  ( 7.999999999999983125, 80.00000000000001421, -9.340760230278089508E-32 ) ) ;
#57528=B_SPLINE_CURVE_WITH_KNOTS ( 'NONE', 3,
 ( #38456, #24027, #43156, #9302, #18413, #37532, #52835, #191, #56603, #8680, #57506, #18722, #28109, #14338, #52519, #27801, #47849, #37852 ),
 .UNSPECIFIED., .F., .F.,
 ( 4, 2, 2, 2, 2, 2, 2, 2, 4 ),
 ( 0.004151178236722271285, 0.004669824733854588579, 0.005188471230986906740, 0.005707117728119224034, 0.006225764225251541328, 0.006744410722383859490, 0.007263057219516176784, 0.007781703716648494945, 0.008300350213780812239 ),
 .UNSPECIFIED. ) ;
#57539=CARTESIAN_POINT ( 'NONE',  ( 53.13317509687642826, 15.49709605010121116, -0.3454668168334632528 ) ) ;
#57569=LINE ( 'NONE', #572, #54937 ) ;
#57637=CARTESIAN_POINT ( 'NONE',  ( 4.999999999999986677, 56.56854249492371878, 56.56854249492391062 ) ) ;
#57712=CARTESIAN_POINT ( 'NONE',  ( 43.00000000000000000, 9.184850993605150311E-15, -75.00000000000001421 ) ) ;
#57746=CYLINDRICAL_SURFACE ( 'NONE', #45683, 75.00000000000001421 ) ;
#57780=CARTESIAN_POINT ( 'NONE',  ( 8.000000000000007105, -56.56854249492410958, 56.56854249492351983 ) ) ;
#57848=AXIS2_PLACEMENT_3D ( 'NONE', #26256, #12806, #31274 ) ;
#57966=CYLINDRICAL_SURFACE ( 'NONE', #915, 2.649999999999992806 ) ;
#57986=VERTEX_POINT ( 'NONE', #54912 ) ;
#58061=AXIS2_PLACEMENT_3D ( 'NONE', #16704, #54892, #31102 ) ;
#58063=CARTESIAN_POINT ( 'NONE',  ( 7.999999999999996447, 2.650000000000832134, -79.99999999999998579 ) ) ;
#58170=CARTESIAN_POINT ( 'NONE',  ( 40.00000000000000000, 0.000000000000000000, 0.000000000000000000 ) ) ;
#58202=CARTESIAN_POINT ( 'NONE',  ( 4.999999999999983125, 80.00000000000001421, -2.649999999999999467 ) ) ;
#58235=PLANE ( 'NONE',  #8569 ) ;
#58266=CARTESIAN_POINT ( 'NONE',  ( 53.01455923075871368, 12.47181771929622585, 0.8542673636581270546 ) ) ;
#58316=CARTESIAN_POINT ( 'NONE',  ( 47.91934067089189142, 12.48479467718134295, 0.6957625760541074067 ) ) ;
#58351=CARTESIAN_POINT ( 'NONE',  ( 8.000000000000012434, -80.00000000000001421, -2.147411887991766662E-31 ) ) ;
#58425=ORIENTED_EDGE ( 'NONE', *, *, #57466, .F. ) ;
#58551=CARTESIAN_POINT ( 'NONE',  ( 7.999999999999986677, 54.69470952478017978, -58.44237546506749226 ) ) ;
#58558=VERTEX_POINT ( 'NONE', #20507 ) ;
#58575=CARTESIAN_POINT ( 'NONE',  ( 53.06478623683360496, 12.48216789012032812, -0.6890828966271237421 ) ) ;
#58662=DIRECTION ( 'NONE',  ( -1.000000000000000000, -1.836909530733573776E-16, 1.925929944387235306E-32 ) ) ;
#58780=DIRECTION ( 'NONE',  ( 1.850371707708593823E-16, -1.000000000000000000, 0.000000000000000000 ) ) ;
#58819=CIRCLE ( 'NONE', #48859, 2.649999999999992806 ) ;
#58894=CARTESIAN_POINT ( 'NONE',  ( 51.67689044586143865, 12.27139102044969654, -2.380666987245603217 ) ) ;
#58931=DIRECTION ( 'NONE',  ( -1.836909530733573776E-16, 1.000000000000000000, 0.000000000000000000 ) ) ;
#58948=AXIS2_PLACEMENT_3D ( 'NONE', #25356, #20057, #30985 ) ;
#59032=ORIENTED_EDGE ( 'NONE', *, *, #40847, .F. ) ;
#59062=DIRECTION ( 'NONE',  ( -1.000000000000000000, -0.000000000000000000, -0.000000000000000000 ) ) ;
#59146=DIRECTION ( 'NONE',  ( -1.000000000000000000, -3.135800716341489291E-16, 1.298891185607901956E-16 ) ) ;
#59319=CARTESIAN_POINT ( 'NONE',  ( 7.999999999999996447, -2.649999999999153033, -80.00000000000004263 ) ) ;
#59327=EDGE_LOOP ( 'NONE', ( #39269, #53240 ) ) ;
#59336=ORIENTED_EDGE ( 'NONE', *, *, #15585, .T. ) ;
#59387=ORIENTED_EDGE ( 'NONE', *, *, #22838, .F. ) ;
#59504=ORIENTED_EDGE ( 'NONE', *, *, #55010, .F. ) ;
#59512=CARTESIAN_POINT ( 'NONE',  ( 53.06478614550846373, 12.48216827162963405, 0.6888196380807342090 ) ) ;
#59558=ORIENTED_EDGE ( 'NONE', *, *, #21221, .T. ) ;
#59605=CYLINDRICAL_SURFACE ( 'NONE', #55471, 2.649999999999997691 ) ;
#59641=ORIENTED_EDGE ( 'NONE', *, *, #23266, .T. ) ;
#59694=DIRECTION ( 'NONE',  ( -1.807003620809173399E-16, 1.000000000000000000, 0.000000000000000000 ) ) ;
#59695=VERTEX_POINT ( 'NONE', #34015 ) ;
#59760=EDGE_CURVE ( 'NONE', #28153, #58558, #30568, .T. ) ;
#59771=AXIS2_PLACEMENT_3D ( 'NONE', #13366, #18683, #33099 ) ;
#59779=CARTESIAN_POINT ( 'NONE',  ( 5.000000000000007994, -54.69470952477976766, 58.44237546506786884 ) ) ;
#59796=VERTEX_POINT ( 'NONE', #13988 ) ;
#59825=DIRECTION ( 'NONE',  ( -1.000000000000000000, -1.836909530733573776E-16, 1.925929944387235853E-32 ) ) ;
#59826=DIRECTION ( 'NONE',  ( -1.000000000000000000, -5.380183451256491399E-17, -1.298891185607892835E-16 ) ) ;
#59853=AXIS2_PLACEMENT_3D ( 'NONE', #54078, #29671, #54384 ) ;
#59860=CARTESIAN_POINT ( 'NONE',  ( 4.999999999999997335, 8.388739760877188892E-13, -80.00000000000001421 ) ) ;
#59918=EDGE_CURVE ( 'NONE', #4178, #9990, #51578, .T. ) ;
#59947=ORIENTED_EDGE ( 'NONE', *, *, #20583, .T. ) ;
#59990=FACE_OUTER_BOUND ( 'NONE', #14654, .T. ) ;
#60027=EDGE_CURVE ( 'NONE', #50598, #1887, #55599, .T. ) ;
#60110=DIRECTION ( 'NONE',  ( -1.000000000000000000, -1.836909530733573776E-16, 1.925929944387235853E-32 ) ) ;
#60160=CARTESIAN_POINT ( 'NONE',  ( 53.14999999999999858, 15.50000000000000711, 1.598617295522242905E-15 ) ) ;
#60244=DIRECTION ( 'NONE',  ( 1.836766033387207149E-16, -1.000000000000000000, 0.000000000000000000 ) ) ;
#60309=PRESENTATION_STYLE_ASSIGNMENT (( #60940 ) ) ;
#60392=DIRECTION ( 'NONE',  ( -3.273063162220391312E-16, 1.000000000000000000, 1.047380211910525220E-14 ) ) ;
#60397=VERTEX_POINT ( 'NONE', #28441 ) ;
#60454=EDGE_CURVE ( 'NONE', #22251, #25443, #37669, .T. ) ;
#60463=CYLINDRICAL_SURFACE ( 'NONE', #61299, 72.00000000000002842 ) ;
#60498=DIRECTION ( 'NONE',  ( -1.000000000000000000, -3.135800716341489291E-16, 1.298891185607901956E-16 ) ) ;
#60513=VECTOR ( 'NONE', #56729, 1000.000000000000000 ) ;
#60559=DIRECTION ( 'NONE',  ( -1.000000000000000000, -1.836909530733573776E-16, 1.925929944387235853E-32 ) ) ;
#60610=VECTOR ( 'NONE', #1654, 1000.000000000000000 ) ;
#60651=VECTOR ( 'NONE', #18007, 1000.000000000000000 ) ;
#60658=DIRECTION ( 'NONE',  ( -1.000000000000000000, -1.836909530733573776E-16, -1.361838123766432833E-32 ) ) ;
#60677=EDGE_CURVE ( 'NONE', #50567, #32701, #31658, .T. ) ;
#60684=FACE_OUTER_BOUND ( 'NONE', #1087, .T. ) ;
#60782=ORIENTED_EDGE ( 'NONE', *, *, #38584, .T. ) ;
#60804=ORIENTED_EDGE ( 'NONE', *, *, #11848, .T. ) ;
#60833=FACE_OUTER_BOUND ( 'NONE', #27122, .T. ) ;
#60848=AXIS2_PLACEMENT_3D ( 'NONE', #17257, #51359, #8444 ) ;
#60854=DIRECTION ( 'NONE',  ( 0.000000000000000000, -0.7071067811865487940, 0.7071067811865461294 ) ) ;
#60856=( GEOMETRIC_REPRESENTATION_CONTEXT ( 3 ) GLOBAL_UNCERTAINTY_ASSIGNED_CONTEXT ( ( #26122 ) ) GLOBAL_UNIT_ASSIGNED_CONTEXT ( ( #60994, #13104, #55363 ) ) REPRESENTATION_CONTEXT ( 'NONE', 'WORKASPACE' ) );
#60857=ORIENTED_EDGE ( 'NONE', *, *, #56910, .T. ) ;
#60864=EDGE_LOOP ( 'NONE', ( #45066, #54673, #33618, #30807 ) ) ;
#60940=SURFACE_STYLE_USAGE ( .BOTH. , #23665 ) ;
#60994=( LENGTH_UNIT ( ) NAMED_UNIT ( * ) SI_UNIT ( .MILLI., .METRE. ) );
#61003=CARTESIAN_POINT ( 'NONE',  ( 7.999999999999981348, 85.00000000000001421, 1.040949779275250495E-14 ) ) ;
#61048=DIRECTION ( 'NONE',  ( 1.000000000000000000, 1.836909530733573776E-16, -1.925929944387235853E-32 ) ) ;
#61061=CARTESIAN_POINT ( 'NONE',  ( 49.64480425791989404, 15.29488547570532297, 2.514152515238056829 ) ) ;
#61064=FACE_OUTER_BOUND ( 'NONE', #19227, .T. ) ;
#61258=ORIENTED_EDGE ( 'NONE', *, *, #45187, .F. ) ;
#61278=CIRCLE ( 'NONE', #7252, 75.00000000000001421 ) ;
#61290=ADVANCED_FACE ( 'NONE', ( #8487 ), #36732, .F. ) ;
#61299=AXIS2_PLACEMENT_3D ( 'NONE', #12895, #55769, #17580 ) ;
#61357=CARTESIAN_POINT ( 'NONE',  ( 50.32685901376226667, 15.27178771460631168, 2.649999999999992806 ) ) ;
#61387=DIRECTION ( 'NONE',  ( 0.000000000000000000, 0.000000000000000000, 1.000000000000000000 ) ) ;
#61439=CARTESIAN_POINT ( 'NONE',  ( 7.999999999999996447, 1.469527624586858429E-15, -1.540743955509788245E-31 ) ) ;
#61452=DIRECTION ( 'NONE',  ( 0.000000000000000000, 1.000000000000000000, 0.000000000000000000 ) ) ;
#61492=DIRECTION ( 'NONE',  ( -1.000000000000000000, -0.000000000000000000, -0.000000000000000000 ) ) ;
#61538=DIRECTION ( 'NONE',  ( -1.000000000000000000, -1.836909530733554547E-16, -1.836909530733573529E-16 ) ) ;
#61572=EDGE_CURVE ( 'NONE', #9990, #4178, #55684, .T. ) ;
#61635=ADVANCED_FACE ( 'NONE', ( #61647 ), #14081, .F. ) ;
#61647=FACE_OUTER_BOUND ( 'NONE', #53558, .T. ) ;
#61651=DIRECTION ( 'NONE',  ( 0.000000000000000000, 0.000000000000000000, -1.000000000000000000 ) ) ;
#61717=ORIENTED_EDGE ( 'NONE', *, *, #6262, .F. ) ;
#61843=EDGE_CURVE ( 'NONE', #16220, #26981, #31791, .T. ) ;
#61857=DIRECTION ( 'NONE',  ( -1.000000000000000000, -1.836909530733573776E-16, 1.361838123766442686E-32 ) ) ;
#61912=CARTESIAN_POINT ( 'NONE',  ( 48.50368771458344952, 15.40123845184989726, -1.751266045669078286 ) ) ;
#61922=ADVANCED_FACE ( 'NONE', ( #1596, #7537 ), #25419, .T. ) ;
#61948=VERTEX_POINT ( 'NONE', #54525 ) ;
ENDSEC;
END-ISO-10303-21;
